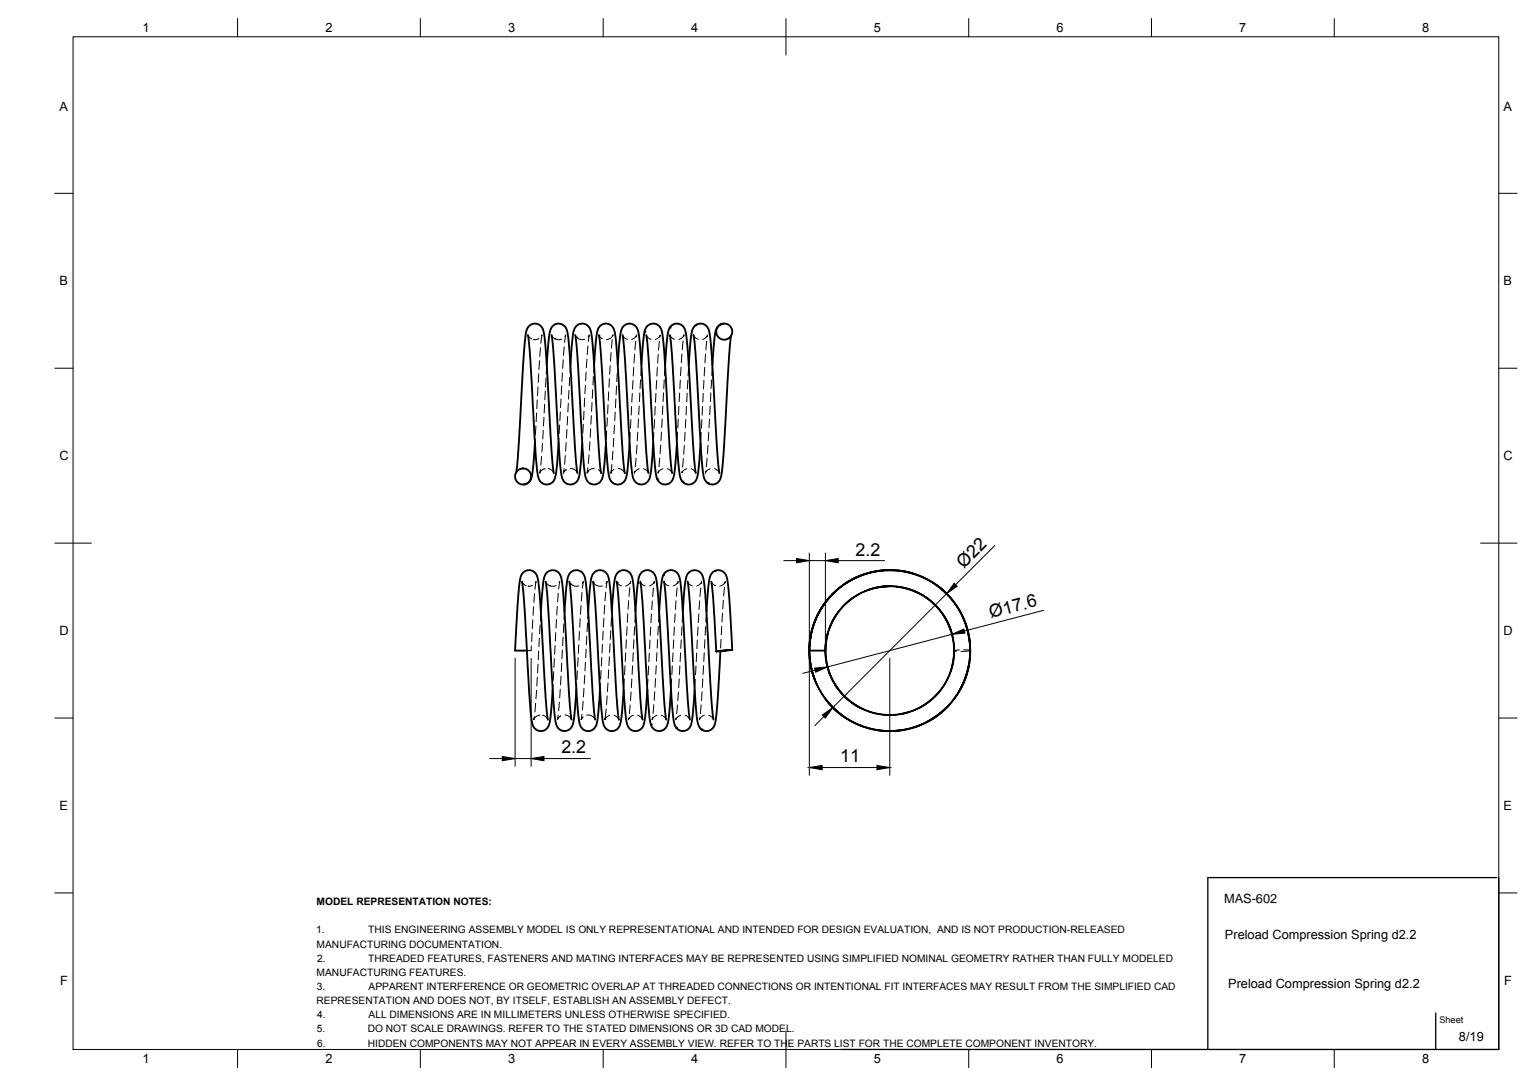
ISO-10303-21;
HEADER;
/* Generated by software containing ST-Developer
 * from STEP Tools, Inc. (www.steptools.com) 
 */

FILE_DESCRIPTION(
/* description */ (''),
/* implementation_level */ '2;1');

FILE_NAME(
/* name */ 'Preload Compression Spring d2.2.step',
/* time_stamp */ '2026-10-15T14:42:47-07:00',
/* author */ (''),
/* organization */ (''),
/* preprocessor_version */ 'ST-DEVELOPER v20.2',
/* originating_system */ 'Autodesk Translation Framework v15.15.0.0',
/* authorisation */ '');

FILE_SCHEMA (('AUTOMOTIVE_DESIGN { 1 0 10303 214 3 1 1 }'));
ENDSEC;

DATA;
#10=MECHANICAL_DESIGN_GEOMETRIC_PRESENTATION_REPRESENTATION('',(#240),#85789);
#204=SHAPE_REPRESENTATION_RELATIONSHIP('SRR','None',#85869,#222);
#222=ADVANCED_BREP_SHAPE_REPRESENTATION('',(#258),#85777);
#240=STYLED_ITEM('',(#85968),#258);
#258=MANIFOLD_SOLID_BREP('Body1',#9887);
#383=B_SPLINE_SURFACE_WITH_KNOTS('',3,3,((#76038,#76039,#76040,#76041,#76042,
#76043,#76044,#76045,#76046,#76047,#76048,#76049,#76050,#76051,#76052,#76053,
#76054,#76055,#76056,#76057,#76058,#76059,#76060,#76061,#76062,#76063,#76064,
#76065,#76066,#76067,#76068,#76069,#76070,#76071,#76072,#76073,#76074,#76075,
#76076,#76077,#76078,#76079,#76080,#76081,#76082,#76083,#76084,#76085,#76086,
#76087,#76088,#76089,#76090,#76091,#76092,#76093,#76094,#76095,#76096,#76097,
#76098,#76099,#76100,#76101,#76102,#76103,#76104,#76105,#76106,#76107,#76108,
#76109,#76110,#76111,#76112,#76113,#76114,#76115,#76116,#76117,#76118,#76119,
#76120,#76121,#76122,#76123,#76124,#76125,#76126,#76127,#76128,#76129,#76130,
#76131,#76132,#76133,#76134,#76135,#76136,#76137,#76138,#76139,#76140,#76141,
#76142,#76143,#76144,#76145,#76146,#76147),(#76148,#76149,#76150,#76151,
#76152,#76153,#76154,#76155,#76156,#76157,#76158,#76159,#76160,#76161,#76162,
#76163,#76164,#76165,#76166,#76167,#76168,#76169,#76170,#76171,#76172,#76173,
#76174,#76175,#76176,#76177,#76178,#76179,#76180,#76181,#76182,#76183,#76184,
#76185,#76186,#76187,#76188,#76189,#76190,#76191,#76192,#76193,#76194,#76195,
#76196,#76197,#76198,#76199,#76200,#76201,#76202,#76203,#76204,#76205,#76206,
#76207,#76208,#76209,#76210,#76211,#76212,#76213,#76214,#76215,#76216,#76217,
#76218,#76219,#76220,#76221,#76222,#76223,#76224,#76225,#76226,#76227,#76228,
#76229,#76230,#76231,#76232,#76233,#76234,#76235,#76236,#76237,#76238,#76239,
#76240,#76241,#76242,#76243,#76244,#76245,#76246,#76247,#76248,#76249,#76250,
#76251,#76252,#76253,#76254,#76255,#76256,#76257),(#76258,#76259,#76260,
#76261,#76262,#76263,#76264,#76265,#76266,#76267,#76268,#76269,#76270,#76271,
#76272,#76273,#76274,#76275,#76276,#76277,#76278,#76279,#76280,#76281,#76282,
#76283,#76284,#76285,#76286,#76287,#76288,#76289,#76290,#76291,#76292,#76293,
#76294,#76295,#76296,#76297,#76298,#76299,#76300,#76301,#76302,#76303,#76304,
#76305,#76306,#76307,#76308,#76309,#76310,#76311,#76312,#76313,#76314,#76315,
#76316,#76317,#76318,#76319,#76320,#76321,#76322,#76323,#76324,#76325,#76326,
#76327,#76328,#76329,#76330,#76331,#76332,#76333,#76334,#76335,#76336,#76337,
#76338,#76339,#76340,#76341,#76342,#76343,#76344,#76345,#76346,#76347,#76348,
#76349,#76350,#76351,#76352,#76353,#76354,#76355,#76356,#76357,#76358,#76359,
#76360,#76361,#76362,#76363,#76364,#76365,#76366,#76367),(#76368,#76369,
#76370,#76371,#76372,#76373,#76374,#76375,#76376,#76377,#76378,#76379,#76380,
#76381,#76382,#76383,#76384,#76385,#76386,#76387,#76388,#76389,#76390,#76391,
#76392,#76393,#76394,#76395,#76396,#76397,#76398,#76399,#76400,#76401,#76402,
#76403,#76404,#76405,#76406,#76407,#76408,#76409,#76410,#76411,#76412,#76413,
#76414,#76415,#76416,#76417,#76418,#76419,#76420,#76421,#76422,#76423,#76424,
#76425,#76426,#76427,#76428,#76429,#76430,#76431,#76432,#76433,#76434,#76435,
#76436,#76437,#76438,#76439,#76440,#76441,#76442,#76443,#76444,#76445,#76446,
#76447,#76448,#76449,#76450,#76451,#76452,#76453,#76454,#76455,#76456,#76457,
#76458,#76459,#76460,#76461,#76462,#76463,#76464,#76465,#76466,#76467,#76468,
#76469,#76470,#76471,#76472,#76473,#76474,#76475,#76476,#76477),(#76478,
#76479,#76480,#76481,#76482,#76483,#76484,#76485,#76486,#76487,#76488,#76489,
#76490,#76491,#76492,#76493,#76494,#76495,#76496,#76497,#76498,#76499,#76500,
#76501,#76502,#76503,#76504,#76505,#76506,#76507,#76508,#76509,#76510,#76511,
#76512,#76513,#76514,#76515,#76516,#76517,#76518,#76519,#76520,#76521,#76522,
#76523,#76524,#76525,#76526,#76527,#76528,#76529,#76530,#76531,#76532,#76533,
#76534,#76535,#76536,#76537,#76538,#76539,#76540,#76541,#76542,#76543,#76544,
#76545,#76546,#76547,#76548,#76549,#76550,#76551,#76552,#76553,#76554,#76555,
#76556,#76557,#76558,#76559,#76560,#76561,#76562,#76563,#76564,#76565,#76566,
#76567,#76568,#76569,#76570,#76571,#76572,#76573,#76574,#76575,#76576,#76577,
#76578,#76579,#76580,#76581,#76582,#76583,#76584,#76585,#76586,#76587),
(#76588,#76589,#76590,#76591,#76592,#76593,#76594,#76595,#76596,#76597,
#76598,#76599,#76600,#76601,#76602,#76603,#76604,#76605,#76606,#76607,#76608,
#76609,#76610,#76611,#76612,#76613,#76614,#76615,#76616,#76617,#76618,#76619,
#76620,#76621,#76622,#76623,#76624,#76625,#76626,#76627,#76628,#76629,#76630,
#76631,#76632,#76633,#76634,#76635,#76636,#76637,#76638,#76639,#76640,#76641,
#76642,#76643,#76644,#76645,#76646,#76647,#76648,#76649,#76650,#76651,#76652,
#76653,#76654,#76655,#76656,#76657,#76658,#76659,#76660,#76661,#76662,#76663,
#76664,#76665,#76666,#76667,#76668,#76669,#76670,#76671,#76672,#76673,#76674,
#76675,#76676,#76677,#76678,#76679,#76680,#76681,#76682,#76683,#76684,#76685,
#76686,#76687,#76688,#76689,#76690,#76691,#76692,#76693,#76694,#76695,#76696,
#76697),(#76698,#76699,#76700,#76701,#76702,#76703,#76704,#76705,#76706,
#76707,#76708,#76709,#76710,#76711,#76712,#76713,#76714,#76715,#76716,#76717,
#76718,#76719,#76720,#76721,#76722,#76723,#76724,#76725,#76726,#76727,#76728,
#76729,#76730,#76731,#76732,#76733,#76734,#76735,#76736,#76737,#76738,#76739,
#76740,#76741,#76742,#76743,#76744,#76745,#76746,#76747,#76748,#76749,#76750,
#76751,#76752,#76753,#76754,#76755,#76756,#76757,#76758,#76759,#76760,#76761,
#76762,#76763,#76764,#76765,#76766,#76767,#76768,#76769,#76770,#76771,#76772,
#76773,#76774,#76775,#76776,#76777,#76778,#76779,#76780,#76781,#76782,#76783,
#76784,#76785,#76786,#76787,#76788,#76789,#76790,#76791,#76792,#76793,#76794,
#76795,#76796,#76797,#76798,#76799,#76800,#76801,#76802,#76803,#76804,#76805,
#76806,#76807),(#76808,#76809,#76810,#76811,#76812,#76813,#76814,#76815,
#76816,#76817,#76818,#76819,#76820,#76821,#76822,#76823,#76824,#76825,#76826,
#76827,#76828,#76829,#76830,#76831,#76832,#76833,#76834,#76835,#76836,#76837,
#76838,#76839,#76840,#76841,#76842,#76843,#76844,#76845,#76846,#76847,#76848,
#76849,#76850,#76851,#76852,#76853,#76854,#76855,#76856,#76857,#76858,#76859,
#76860,#76861,#76862,#76863,#76864,#76865,#76866,#76867,#76868,#76869,#76870,
#76871,#76872,#76873,#76874,#76875,#76876,#76877,#76878,#76879,#76880,#76881,
#76882,#76883,#76884,#76885,#76886,#76887,#76888,#76889,#76890,#76891,#76892,
#76893,#76894,#76895,#76896,#76897,#76898,#76899,#76900,#76901,#76902,#76903,
#76904,#76905,#76906,#76907,#76908,#76909,#76910,#76911,#76912,#76913,#76914,
#76915,#76916,#76917),(#76918,#76919,#76920,#76921,#76922,#76923,#76924,
#76925,#76926,#76927,#76928,#76929,#76930,#76931,#76932,#76933,#76934,#76935,
#76936,#76937,#76938,#76939,#76940,#76941,#76942,#76943,#76944,#76945,#76946,
#76947,#76948,#76949,#76950,#76951,#76952,#76953,#76954,#76955,#76956,#76957,
#76958,#76959,#76960,#76961,#76962,#76963,#76964,#76965,#76966,#76967,#76968,
#76969,#76970,#76971,#76972,#76973,#76974,#76975,#76976,#76977,#76978,#76979,
#76980,#76981,#76982,#76983,#76984,#76985,#76986,#76987,#76988,#76989,#76990,
#76991,#76992,#76993,#76994,#76995,#76996,#76997,#76998,#76999,#77000,#77001,
#77002,#77003,#77004,#77005,#77006,#77007,#77008,#77009,#77010,#77011,#77012,
#77013,#77014,#77015,#77016,#77017,#77018,#77019,#77020,#77021,#77022,#77023,
#77024,#77025,#77026,#77027),(#77028,#77029,#77030,#77031,#77032,#77033,
#77034,#77035,#77036,#77037,#77038,#77039,#77040,#77041,#77042,#77043,#77044,
#77045,#77046,#77047,#77048,#77049,#77050,#77051,#77052,#77053,#77054,#77055,
#77056,#77057,#77058,#77059,#77060,#77061,#77062,#77063,#77064,#77065,#77066,
#77067,#77068,#77069,#77070,#77071,#77072,#77073,#77074,#77075,#77076,#77077,
#77078,#77079,#77080,#77081,#77082,#77083,#77084,#77085,#77086,#77087,#77088,
#77089,#77090,#77091,#77092,#77093,#77094,#77095,#77096,#77097,#77098,#77099,
#77100,#77101,#77102,#77103,#77104,#77105,#77106,#77107,#77108,#77109,#77110,
#77111,#77112,#77113,#77114,#77115,#77116,#77117,#77118,#77119,#77120,#77121,
#77122,#77123,#77124,#77125,#77126,#77127,#77128,#77129,#77130,#77131,#77132,
#77133,#77134,#77135,#77136,#77137)),.UNSPECIFIED.,.T.,.F.,.F.,(4,1,1,1,
1,1,1,4),(4,1,1,1,1,1,1,1,1,1,1,1,1,1,1,1,1,1,1,1,1,1,1,1,1,1,1,1,1,1,1,
1,1,1,1,1,1,1,1,1,1,1,1,1,1,1,1,1,1,1,1,1,1,1,1,1,1,1,1,1,1,1,1,1,1,1,1,
1,1,1,1,1,1,1,1,1,1,1,1,1,1,1,1,1,1,1,1,1,1,1,1,1,1,1,1,1,1,1,1,1,1,1,1,
1,1,1,1,4),(-3.14159265358979,-2.24399475256414,-1.34639685153848,-0.448798950512828,
0.448798950512828,1.34639685153848,2.24399475256414,3.14159265358979),(0.,
0.00446428571428571,0.00892857142857143,0.0178571428571429,0.0267857142857143,
0.0357142857142857,0.0446428571428571,0.0535714285714286,0.0625,0.0714285714285714,
0.0803571428571428,0.0892857142857143,0.0982142857142857,0.107142857142857,
0.116071428571429,0.125,0.133928571428571,0.142857142857143,0.154761904761905,
0.166666666666667,0.178571428571429,0.18452380952381,0.19047619047619,0.196428571428571,
0.202380952380952,0.214285714285714,0.222222222222222,0.23015873015873,
0.238095238095238,0.244047619047619,0.25,0.261904761904762,0.273809523809524,
0.285714285714286,0.297619047619048,0.30952380952381,0.321428571428571,
0.333333333333333,0.341269841269841,0.349206349206349,0.357142857142857,
0.365079365079365,0.373015873015873,0.380952380952381,0.392857142857143,
0.404761904761905,0.416666666666667,0.428571428571429,0.44047619047619,
0.452380952380952,0.46031746031746,0.468253968253968,0.472222222222222,
0.476190476190476,0.486772486772487,0.492063492063492,0.5,0.507936507936508,
0.515873015873016,0.523809523809524,0.535714285714286,0.547619047619048,
0.55952380952381,0.571428571428571,0.583333333333333,0.595238095238095,
0.607142857142857,0.619047619047619,0.626984126984127,0.634920634920635,
0.642857142857143,0.650793650793651,0.658730158730159,0.666666666666667,
0.674603174603175,0.682539682539683,0.69047619047619,0.702380952380952,
0.714285714285714,0.726190476190476,0.738095238095238,0.75,0.761904761904762,
0.773809523809524,0.785714285714286,0.797619047619047,0.809523809523809,
0.821428571428571,0.833333333333333,0.845238095238095,0.857142857142857,
0.866071428571429,0.875,0.883928571428571,0.892857142857143,0.901785714285714,
0.910714285714286,0.919642857142857,0.928571428571429,0.9375,0.946428571428571,
0.955357142857143,0.964285714285714,0.973214285714286,0.982142857142857,
0.991071428571429,0.995535714285714,1.),.UNSPECIFIED.);
#905=B_SPLINE_CURVE_WITH_KNOTS('',3,(#77139,#77140,#77141,#77142,#77143,
#77144,#77145,#77146,#77147,#77148,#77149,#77150,#77151,#77152,#77153,#77154,
#77155,#77156,#77157,#77158,#77159,#77160,#77161,#77162,#77163,#77164,#77165,
#77166,#77167,#77168,#77169,#77170,#77171,#77172,#77173,#77174,#77175,#77176),
 .UNSPECIFIED.,.T.,.F.,(4,2,2,2,2,2,2,2,2,2,2,2,2,2,2,2,2,2,4),(-0.605125399548974,
-0.601986519691417,-0.572296417272211,-0.544506901286991,-0.51205526449825,
-0.473980307125887,-0.436263250016685,-0.397515325089208,-0.367226247639718,
-0.338720455098409,-0.30995049023698,-0.27886558943038,-0.238746391927005,
-0.193651773165657,-0.137323097666455,-0.0888290194031273,-0.0473891574083154,
-0.00368586125467713,0.),.UNSPECIFIED.);
#906=B_SPLINE_CURVE_WITH_KNOTS('',3,(#77178,#77179,#77180,#77181,#77182,
#77183,#77184,#77185,#77186,#77187,#77188,#77189,#77190,#77191,#77192,#77193,
#77194,#77195,#77196,#77197,#77198,#77199,#77200,#77201,#77202,#77203,#77204,
#77205,#77206,#77207,#77208,#77209,#77210,#77211,#77212,#77213,#77214,#77215,
#77216,#77217,#77218,#77219,#77220,#77221,#77222,#77223,#77224,#77225,#77226,
#77227,#77228,#77229,#77230,#77231,#77232,#77233,#77234,#77235,#77236,#77237,
#77238,#77239,#77240,#77241,#77242,#77243,#77244,#77245,#77246,#77247,#77248,
#77249,#77250,#77251,#77252,#77253,#77254,#77255,#77256,#77257,#77258,#77259,
#77260,#77261,#77262,#77263,#77264,#77265,#77266,#77267,#77268,#77269,#77270,
#77271,#77272,#77273,#77274,#77275,#77276,#77277,#77278,#77279,#77280,#77281,
#77282,#77283,#77284,#77285,#77286,#77287),.UNSPECIFIED.,.F.,.F.,(4,1,1,
1,1,1,1,1,1,1,1,1,1,1,1,1,1,1,1,1,1,1,1,1,1,1,1,1,1,1,1,1,1,1,1,1,1,1,1,
1,1,1,1,1,1,1,1,1,1,1,1,1,1,1,1,1,1,1,1,1,1,1,1,1,1,1,1,1,1,1,1,1,1,1,1,
1,1,1,1,1,1,1,1,1,1,1,1,1,1,1,1,1,1,1,1,1,1,1,1,1,1,1,1,1,1,1,1,4),(0.,
0.00446428571428571,0.00892857142857143,0.0178571428571429,0.0267857142857143,
0.0357142857142857,0.0446428571428571,0.0535714285714286,0.0625,0.0714285714285714,
0.0803571428571428,0.0892857142857143,0.0982142857142857,0.107142857142857,
0.116071428571429,0.125,0.133928571428571,0.142857142857143,0.154761904761905,
0.166666666666667,0.178571428571429,0.18452380952381,0.19047619047619,0.196428571428571,
0.202380952380952,0.214285714285714,0.222222222222222,0.23015873015873,
0.238095238095238,0.244047619047619,0.25,0.261904761904762,0.273809523809524,
0.285714285714286,0.297619047619048,0.30952380952381,0.321428571428571,
0.333333333333333,0.341269841269841,0.349206349206349,0.357142857142857,
0.365079365079365,0.373015873015873,0.380952380952381,0.392857142857143,
0.404761904761905,0.416666666666667,0.428571428571429,0.44047619047619,
0.452380952380952,0.46031746031746,0.468253968253968,0.472222222222222,
0.476190476190476,0.486772486772487,0.492063492063492,0.5,0.507936507936508,
0.515873015873016,0.523809523809524,0.535714285714286,0.547619047619048,
0.55952380952381,0.571428571428571,0.583333333333333,0.595238095238095,
0.607142857142857,0.619047619047619,0.626984126984127,0.634920634920635,
0.642857142857143,0.650793650793651,0.658730158730159,0.666666666666667,
0.674603174603175,0.682539682539683,0.69047619047619,0.702380952380952,
0.714285714285714,0.726190476190476,0.738095238095238,0.75,0.761904761904762,
0.773809523809524,0.785714285714286,0.797619047619047,0.809523809523809,
0.821428571428571,0.833333333333333,0.845238095238095,0.857142857142857,
0.866071428571429,0.875,0.883928571428571,0.892857142857143,0.901785714285714,
0.910714285714286,0.919642857142857,0.928571428571429,0.9375,0.946428571428571,
0.955357142857143,0.964285714285714,0.973214285714286,0.982142857142857,
0.991071428571429,0.995535714285714,1.),.UNSPECIFIED.);
#907=B_SPLINE_CURVE_WITH_KNOTS('',3,(#77288,#77289,#77290,#77291,#77292,
#77293,#77294,#77295,#77296,#77297,#77298,#77299,#77300,#77301,#77302,#77303,
#77304,#77305,#77306,#77307,#77308,#77309,#77310,#77311,#77312,#77313,#77314,
#77315,#77316,#77317,#77318,#77319,#77320,#77321,#77322,#77323,#77324,#77325),
 .UNSPECIFIED.,.T.,.F.,(4,2,2,2,2,2,2,2,2,2,2,2,2,2,2,2,2,2,4),(-0.605125399680566,
-0.601986519826148,-0.572296417399655,-0.544506901407513,-0.512055264610774,
-0.473980307229046,-0.436263250110675,-0.397515325173783,-0.367226247717055,
-0.338720455168909,-0.309950490300473,-0.278865589486237,-0.238746391973086,
-0.1936517732017,-0.137323097692225,-0.0888290194200642,-0.0473891574177423,
-0.00368586125594956,0.),.UNSPECIFIED.);
#1110=PLANE('',#10563);
#1111=PLANE('',#10564);
#2712=FACE_OUTER_BOUND('',#3276,.T.);
#2713=FACE_OUTER_BOUND('',#3277,.T.);
#2714=FACE_OUTER_BOUND('',#3278,.T.);
#3276=EDGE_LOOP('',(#8405,#8406,#8407,#8408));
#3277=EDGE_LOOP('',(#8409));
#3278=EDGE_LOOP('',(#8410));
#4601=VERTEX_POINT('',#77138);
#4602=VERTEX_POINT('',#77177);
#5930=EDGE_CURVE('',#4601,#4601,#905,.T.);
#5931=EDGE_CURVE('',#4601,#4602,#906,.T.);
#5932=EDGE_CURVE('',#4602,#4602,#907,.T.);
#8405=ORIENTED_EDGE('',*,*,#5930,.T.);
#8406=ORIENTED_EDGE('',*,*,#5931,.T.);
#8407=ORIENTED_EDGE('',*,*,#5932,.F.);
#8408=ORIENTED_EDGE('',*,*,#5931,.F.);
#8409=ORIENTED_EDGE('',*,*,#5932,.T.);
#8410=ORIENTED_EDGE('',*,*,#5930,.F.);
#9690=ADVANCED_FACE('',(#2712),#383,.T.);
#9691=ADVANCED_FACE('',(#2713),#1110,.T.);
#9692=ADVANCED_FACE('',(#2714),#1111,.F.);
#9887=CLOSED_SHELL('',(#9690,#9691,#9692));
#10562=AXIS2_PLACEMENT_3D('',#76037,#12217,#12218);
#10563=AXIS2_PLACEMENT_3D('',#77326,#12219,#12220);
#10564=AXIS2_PLACEMENT_3D('',#77327,#12221,#12222);
#12217=DIRECTION('axis',(0.,0.,1.));
#12218=DIRECTION('refdir',(1.,0.,0.));
#12219=DIRECTION('center_axis',(-0.0185160100832464,-0.994867197984037,
0.0994807305260099));
#12220=DIRECTION('ref_axis',(0.933205561217733,0.0185160101174801,0.358865626497753));
#12221=DIRECTION('center_axis',(0.,1.,0.));
#12222=DIRECTION('ref_axis',(1.,0.,0.));
#76037=CARTESIAN_POINT('',(0.,0.,0.));
#76038=CARTESIAN_POINT('Ctrl Pts',(0.88,2.1,9.525));
#76039=CARTESIAN_POINT('Ctrl Pts',(0.879914606625585,2.17110785049955,9.52865476385635));
#76040=CARTESIAN_POINT('Ctrl Pts',(0.863232117186907,2.3095104036224,9.53591397312323));
#76041=CARTESIAN_POINT('Ctrl Pts',(0.7646146646842,2.57432753790838,9.55048599717583));
#76042=CARTESIAN_POINT('Ctrl Pts',(0.52875066403414,2.8457083400553,9.56867094599734));
#76043=CARTESIAN_POINT('Ctrl Pts',(0.127238756664634,3.00552936974926,9.59051359518968));
#76044=CARTESIAN_POINT('Ctrl Pts',(-0.302716205619033,2.96306288294985,
9.61235380295566));
#76045=CARTESIAN_POINT('Ctrl Pts',(-0.665427657999688,2.72799341501097,
9.63420407641812));
#76046=CARTESIAN_POINT('Ctrl Pts',(-0.879826065415376,2.3524940033895,9.65606121698024));
#76047=CARTESIAN_POINT('Ctrl Pts',(-0.89799221853441,1.92029343459682,9.67792905414005));
#76048=CARTESIAN_POINT('Ctrl Pts',(-0.715657796510551,1.52775201761214,
9.69980826165769));
#76049=CARTESIAN_POINT('Ctrl Pts',(-0.37329244035757,1.26252484692041,9.72170089413125));
#76050=CARTESIAN_POINT('Ctrl Pts',(0.0529042162174613,1.18397194405211,
9.7436083723133));
#76051=CARTESIAN_POINT('Ctrl Pts',(0.467926525737336,1.30987826775351,9.76553239226868));
#76052=CARTESIAN_POINT('Ctrl Pts',(0.77911594458734,1.61250328722602,9.78747453406851));
#76053=CARTESIAN_POINT('Ctrl Pts',(0.916833254715888,2.02450810034898,9.8094364412056));
#76054=CARTESIAN_POINT('Ctrl Pts',(0.84999015619955,2.45432327019144,9.83141968646686));
#76055=CARTESIAN_POINT('Ctrl Pts',(0.593134887517594,2.80556810401153,9.85342584950507));
#76056=CARTESIAN_POINT('Ctrl Pts',(0.159785468035136,3.02235194398505,9.87790429996245));
#76057=CARTESIAN_POINT('Ctrl Pts',(-0.382738476891779,2.97204316801605,
9.90486768286448));
#76058=CARTESIAN_POINT('Ctrl Pts',(-0.827943575417754,2.57464859578558,
9.93433214776037));
#76059=CARTESIAN_POINT('Ctrl Pts',(-0.928540642244484,2.0879125901631,9.95893043030863));
#76060=CARTESIAN_POINT('Ctrl Pts',(-0.82506221727755,1.71823863855703,9.97863755083128));
#76061=CARTESIAN_POINT('Ctrl Pts',(-0.665238898770628,1.47861418311032,
9.99343255715118));
#76062=CARTESIAN_POINT('Ctrl Pts',(-0.438025190317537,1.3012081221325,10.0082426633322));
#76063=CARTESIAN_POINT('Ctrl Pts',(-0.0759140953759721,1.16989403941721,
10.0280101634631));
#76064=CARTESIAN_POINT('Ctrl Pts',(0.353590617267489,1.22647296601624,10.0494595111079));
#76065=CARTESIAN_POINT('Ctrl Pts',(0.71282299611785,1.50640456177768,10.0726022736917));
#76066=CARTESIAN_POINT('Ctrl Pts',(0.895311256816217,1.85157831854142,10.0924697020734));
#76067=CARTESIAN_POINT('Ctrl Pts',(0.917661293713379,2.20976194577009,10.1107106042816));
#76068=CARTESIAN_POINT('Ctrl Pts',(0.819212469046223,2.51761130734418,10.127317066638));
#76069=CARTESIAN_POINT('Ctrl Pts',(0.591924394917487,2.83289082559773,10.1472698428113));
#76070=CARTESIAN_POINT('Ctrl Pts',(0.141288805504938,3.06103897732418,10.172258699084));
#76071=CARTESIAN_POINT('Ctrl Pts',(-0.458527011040082,2.95925151709148,
10.2023249565719));
#76072=CARTESIAN_POINT('Ctrl Pts',(-0.88162766536303,2.52027411449529,10.2324736532743));
#76073=CARTESIAN_POINT('Ctrl Pts',(-0.961653185964405,1.91393657438503,
10.2627077273853));
#76074=CARTESIAN_POINT('Ctrl Pts',(-0.665231767857691,1.37715957803001,
10.2930297792945));
#76075=CARTESIAN_POINT('Ctrl Pts',(-0.105988685338195,1.12026073865136,
10.3234425669733));
#76076=CARTESIAN_POINT('Ctrl Pts',(0.430538820721984,1.23255710504194,10.3505590141325));
#76077=CARTESIAN_POINT('Ctrl Pts',(0.777157271318668,1.54704609431923,10.3743479205533));
#76078=CARTESIAN_POINT('Ctrl Pts',(0.937973646848606,1.91510656924282,10.3947816504623));
#76079=CARTESIAN_POINT('Ctrl Pts',(0.932931736507626,2.31778957988939,10.4152592321293));
#76080=CARTESIAN_POINT('Ctrl Pts',(0.762578582228501,2.68366310973811,10.4357813746755));
#76081=CARTESIAN_POINT('Ctrl Pts',(0.455963235969408,2.94715653506223,10.4563486739678));
#76082=CARTESIAN_POINT('Ctrl Pts',(0.00240142086611935,3.08166579400621,
10.480397254692));
#76083=CARTESIAN_POINT('Ctrl Pts',(-0.538455390507358,2.94820992747045,
10.5079586157699));
#76084=CARTESIAN_POINT('Ctrl Pts',(-0.940666416691817,2.46401744657124,
10.5390713811047));
#76085=CARTESIAN_POINT('Ctrl Pts',(-0.976029443563649,1.83335883304997,
10.5702921359498));
#76086=CARTESIAN_POINT('Ctrl Pts',(-0.629306856593687,1.30317046301086,
10.6016225477596));
#76087=CARTESIAN_POINT('Ctrl Pts',(-0.0328763589810331,1.08144514613719,
10.6330641573791));
#76088=CARTESIAN_POINT('Ctrl Pts',(0.511901871764286,1.23876013099839,10.6611123163153));
#76089=CARTESIAN_POINT('Ctrl Pts',(0.845208777494887,1.59002857501027,10.6857282761483));
#76090=CARTESIAN_POINT('Ctrl Pts',(0.959937391714928,1.91692164410815,10.7033535735637));
#76091=CARTESIAN_POINT('Ctrl Pts',(0.964709509971458,2.19002072343591,10.7174794574177));
#76092=CARTESIAN_POINT('Ctrl Pts',(0.903969607200192,2.50338072207659,10.7339796596208));
#76093=CARTESIAN_POINT('Ctrl Pts',(0.708976511873778,2.79903473649909,10.7516978643424));
#76094=CARTESIAN_POINT('Ctrl Pts',(0.359111666410103,3.02058677865832,10.7730116718645));
#76095=CARTESIAN_POINT('Ctrl Pts',(-0.0055195068732309,3.09939687665217,
10.7919958841582));
#76096=CARTESIAN_POINT('Ctrl Pts',(-0.417331250225881,3.01093271757532,
10.8134054790171));
#76097=CARTESIAN_POINT('Ctrl Pts',(-0.756608961158023,2.76032613000462,
10.8348676292604));
#76098=CARTESIAN_POINT('Ctrl Pts',(-0.998865593098056,2.33000290793379,
10.8599683150449));
#76099=CARTESIAN_POINT('Ctrl Pts',(-0.988791187924089,1.74845036869023,
10.8887429491342));
#76100=CARTESIAN_POINT('Ctrl Pts',(-0.588714669350558,1.22669384301482,
10.9212338011637));
#76101=CARTESIAN_POINT('Ctrl Pts',(0.044909234496707,1.04388405761621,10.9538443040117));
#76102=CARTESIAN_POINT('Ctrl Pts',(0.665762350574508,1.27382859359802,10.9865746011287));
#76103=CARTESIAN_POINT('Ctrl Pts',(1.02994927065475,1.82963242200099,11.0194247010519));
#76104=CARTESIAN_POINT('Ctrl Pts',(0.99292771913683,2.49532007970257,11.0523944801788));
#76105=CARTESIAN_POINT('Ctrl Pts',(0.566047404042377,3.01118540039736,11.0854836852924));
#76106=CARTESIAN_POINT('Ctrl Pts',(-0.0131656805453273,3.1545072720966,
11.1150021335127));
#76107=CARTESIAN_POINT('Ctrl Pts',(-0.501834747536299,3.00971245930524,
11.1409075995603));
#76108=CARTESIAN_POINT('Ctrl Pts',(-0.833654637909307,2.72466132918788,
11.1631647757637));
#76109=CARTESIAN_POINT('Ctrl Pts',(-1.01904932840502,2.32688792491809,11.1854742337572));
#76110=CARTESIAN_POINT('Ctrl Pts',(-1.0247320303861,1.8873087550975,11.2078357472338));
#76111=CARTESIAN_POINT('Ctrl Pts',(-0.848433071641297,1.48323440703255,
11.2302490424206));
#76112=CARTESIAN_POINT('Ctrl Pts',(-0.5209916303453,1.18686010809674,11.2527138516101));
#76113=CARTESIAN_POINT('Ctrl Pts',(-0.0994474829318688,1.05086828612434,
11.2752298585268));
#76114=CARTESIAN_POINT('Ctrl Pts',(0.341286571712092,1.10081439784123,11.297796723956));
#76115=CARTESIAN_POINT('Ctrl Pts',(0.787934060544661,1.36522529701193,11.3241836591263));
#76116=CARTESIAN_POINT('Ctrl Pts',(1.08440822726537,1.89981767692546,11.3544236935599));
#76117=CARTESIAN_POINT('Ctrl Pts',(0.99437189083192,2.58466520846377,11.3885550724356));
#76118=CARTESIAN_POINT('Ctrl Pts',(0.51422832678732,3.08343949927552,11.4227963300144));
#76119=CARTESIAN_POINT('Ctrl Pts',(-0.170956362315584,3.20042729316684,
11.4571457685877));
#76120=CARTESIAN_POINT('Ctrl Pts',(-0.792809143568463,2.88603885152724,
11.49160167588));
#76121=CARTESIAN_POINT('Ctrl Pts',(-1.10815562220614,2.26212033857722,11.5261621918766));
#76122=CARTESIAN_POINT('Ctrl Pts',(-0.990980784814367,1.57098681332194,
11.5608252913622));
#76123=CARTESIAN_POINT('Ctrl Pts',(-0.484736723033935,1.08260154598769,
11.5955889188738));
#76124=CARTESIAN_POINT('Ctrl Pts',(0.214307763377102,0.991032096532327,
11.6304507824074));
#76125=CARTESIAN_POINT('Ctrl Pts',(0.833298379906107,1.33271197734595,11.6654086518246));
#76126=CARTESIAN_POINT('Ctrl Pts',(1.12908711130714,1.97705558535849,11.7004600148669));
#76127=CARTESIAN_POINT('Ctrl Pts',(0.984170425255086,2.67277304384029,11.7356024461146));
#76128=CARTESIAN_POINT('Ctrl Pts',(0.452808643636702,3.14802102155422,11.7708333087139));
#76129=CARTESIAN_POINT('Ctrl Pts',(-0.198836507924274,3.20872213800758,
11.8032068201948));
#76130=CARTESIAN_POINT('Ctrl Pts',(-0.720833985617695,2.9475724124579,11.8326976979388));
#76131=CARTESIAN_POINT('Ctrl Pts',(-1.03122512713103,2.52323917223077,11.8592848682016));
#76132=CARTESIAN_POINT('Ctrl Pts',(-1.11221371795246,2.00254397936835,11.8859162010712));
#76133=CARTESIAN_POINT('Ctrl Pts',(-0.944978677865563,1.50212478400673,
11.9125904181942));
#76134=CARTESIAN_POINT('Ctrl Pts',(-0.566096651435205,1.13364169683645,
11.9393062323883));
#76135=CARTESIAN_POINT('Ctrl Pts',(-0.0596069971212731,0.97996909355213,
11.966062281935));
#76136=CARTESIAN_POINT('Ctrl Pts',(0.461675051948685,1.07603593590851,11.9928572469173));
#76137=CARTESIAN_POINT('Ctrl Pts',(0.88129231323125,1.40110770643291,12.0196896905075));
#76138=CARTESIAN_POINT('Ctrl Pts',(1.10519737818586,1.88315811002375,12.0465583931276));
#76139=CARTESIAN_POINT('Ctrl Pts',(1.08283365883886,2.41488670097258,12.0734615789711));
#76140=CARTESIAN_POINT('Ctrl Pts',(0.818591168747924,2.87760074176854,12.100398642491));
#76141=CARTESIAN_POINT('Ctrl Pts',(0.370893737846914,3.16774776724325,12.1273662612715));
#76142=CARTESIAN_POINT('Ctrl Pts',(-0.160578831483255,3.22009488317826,
12.154367120808));
#76143=CARTESIAN_POINT('Ctrl Pts',(-0.657438304412148,3.02243699025829,
12.181390412703));
#76144=CARTESIAN_POINT('Ctrl Pts',(-0.949764066307816,2.68573447988004,
12.2039450357004));
#76145=CARTESIAN_POINT('Ctrl Pts',(-1.07182425162092,2.35796849387404,12.2219800536891));
#76146=CARTESIAN_POINT('Ctrl Pts',(-1.09256785760649,2.18550272007321,12.2310256553714));
#76147=CARTESIAN_POINT('Ctrl Pts',(-1.09265261173395,2.09796323888708,12.2355247810852));
#76148=CARTESIAN_POINT('Ctrl Pts',(0.88,2.1,9.55791192303761));
#76149=CARTESIAN_POINT('Ctrl Pts',(0.879783916285541,2.17106190544998,9.56156549634868));
#76150=CARTESIAN_POINT('Ctrl Pts',(0.862819487639945,2.30936028696044,9.56882270408062));
#76151=CARTESIAN_POINT('Ctrl Pts',(0.763769645522231,2.57374536624056,9.58338184659129));
#76152=CARTESIAN_POINT('Ctrl Pts',(0.527681439909107,2.84421258618503,9.60154403506069));
#76153=CARTESIAN_POINT('Ctrl Pts',(0.126836189332554,3.00282054305338,9.6233360843192));
#76154=CARTESIAN_POINT('Ctrl Pts',(-0.301578089003487,2.9596327314869,9.64510671305593));
#76155=CARTESIAN_POINT('Ctrl Pts',(-0.662248104445556,2.72485823025643,
9.66686668449843));
#76156=CARTESIAN_POINT('Ctrl Pts',(-0.87477101414986,2.35090800902427,9.68861370251383));
#76157=CARTESIAN_POINT('Ctrl Pts',(-0.891962086690084,1.92134378925048,
9.71035132236448));
#76158=CARTESIAN_POINT('Ctrl Pts',(-0.71013501547485,1.53195117584763,9.73208047576603));
#76159=CARTESIAN_POINT('Ctrl Pts',(-0.369972269812193,1.2695301574022,9.75380324748816));
#76160=CARTESIAN_POINT('Ctrl Pts',(0.0525992830413849,1.19253118829567,
9.77552119527361));
#76161=CARTESIAN_POINT('Ctrl Pts',(0.463319878103491,1.31804354326137,9.79723612745198));
#76162=CARTESIAN_POINT('Ctrl Pts',(0.770594784068131,1.61807714145974,9.81894973497212));
#76163=CARTESIAN_POINT('Ctrl Pts',(0.90590391628519,2.02562383372829,9.84066384510364));
#76164=CARTESIAN_POINT('Ctrl Pts',(0.839026217634196,2.44999742219886,9.86238006152402));
#76165=CARTESIAN_POINT('Ctrl Pts',(0.584857943541199,2.79609540610752,9.88410036302005));
#76166=CARTESIAN_POINT('Ctrl Pts',(0.15715540696274,3.00896823215133,9.90823975031835));
#76167=CARTESIAN_POINT('Ctrl Pts',(-0.377152993385563,2.95829410746318,
9.93480658955309));
#76168=CARTESIAN_POINT('Ctrl Pts',(-0.814397042063615,2.56634291336892,
9.96380668194593));
#76169=CARTESIAN_POINT('Ctrl Pts',(-0.912281798203633,2.08773618372905,
9.9879885560003));
#76170=CARTESIAN_POINT('Ctrl Pts',(-0.80994027967792,1.72488593264374,10.007344749781));
#76171=CARTESIAN_POINT('Ctrl Pts',(-0.652597501593231,1.48997710639104,
10.0218694825692));
#76172=CARTESIAN_POINT('Ctrl Pts',(-0.429334265664847,1.31636286686092,
10.036401726932));
#76173=CARTESIAN_POINT('Ctrl Pts',(-0.0739971908554309,1.18829325899891,
10.0557871102574));
#76174=CARTESIAN_POINT('Ctrl Pts',(0.346806406792938,1.24460770613069,10.0768146985648));
#76175=CARTESIAN_POINT('Ctrl Pts',(0.697974642411667,1.51937892964619,10.0994750183564));
#76176=CARTESIAN_POINT('Ctrl Pts',(0.87586983164938,1.85746669220029,10.1189161511382));
#76177=CARTESIAN_POINT('Ctrl Pts',(0.897034042189538,2.20777551093713,10.1367564439922));
#76178=CARTESIAN_POINT('Ctrl Pts',(0.800234096584245,2.5084630157536,10.152988370211));
#76179=CARTESIAN_POINT('Ctrl Pts',(0.577596139139017,2.81603174879275,10.1724819296167));
#76180=CARTESIAN_POINT('Ctrl Pts',(0.137179583427464,3.03788753933788,10.1968844302235));
#76181=CARTESIAN_POINT('Ctrl Pts',(-0.447719726782846,2.93741039885078,
10.2262174469579));
#76182=CARTESIAN_POINT('Ctrl Pts',(-0.8592452583341,2.50872159304617,10.2556077729931));
#76183=CARTESIAN_POINT('Ctrl Pts',(-0.935997001543472,1.91804036079765,
10.2850576889373));
#76184=CARTESIAN_POINT('Ctrl Pts',(-0.646471737706749,1.3962267816677,10.3145716941238));
#76185=CARTESIAN_POINT('Ctrl Pts',(-0.102097088466362,1.14747264463815,
10.3441525825305));
#76186=CARTESIAN_POINT('Ctrl Pts',(0.419131076191686,1.25764685588435,10.3705107921544));
#76187=CARTESIAN_POINT('Ctrl Pts',(0.755233370608568,1.56377441619041,10.3936200727939));
#76188=CARTESIAN_POINT('Ctrl Pts',(0.910698712173214,1.92145284521483,10.4134626290806));
#76189=CARTESIAN_POINT('Ctrl Pts',(0.905060795811563,2.3122898350333,10.433339759045));
#76190=CARTESIAN_POINT('Ctrl Pts',(0.739099621706325,2.66695860331452,10.453252117855));
#76191=CARTESIAN_POINT('Ctrl Pts',(0.441230372512847,2.92195825542685,10.4732014482075));
#76192=CARTESIAN_POINT('Ctrl Pts',(0.00121674788033055,3.05154102121814,
10.4965196435521));
#76193=CARTESIAN_POINT('Ctrl Pts',(-0.522748489859997,2.92119140764988,
10.5232357617401));
#76194=CARTESIAN_POINT('Ctrl Pts',(-0.911497386825926,2.45137002542038,
10.5533776932785));
#76195=CARTESIAN_POINT('Ctrl Pts',(-0.944589337394057,1.84057261493696,
10.5836150456035));
#76196=CARTESIAN_POINT('Ctrl Pts',(-0.607970601887274,1.32795366098775,
10.6139463426483));
#76197=CARTESIAN_POINT('Ctrl Pts',(-0.0303722616549957,1.11446027835103,
10.6443758271437));
#76198=CARTESIAN_POINT('Ctrl Pts',(0.496414421501777,1.26764280902697,10.6715139458982));
#76199=CARTESIAN_POINT('Ctrl Pts',(0.818195108939898,1.60801290269984,10.6953251867043));
#76200=CARTESIAN_POINT('Ctrl Pts',(0.928577482097722,1.92437513921087,10.7123719721017));
#76201=CARTESIAN_POINT('Ctrl Pts',(0.932712814366555,2.18849028957719,10.7260329283826));
#76202=CARTESIAN_POINT('Ctrl Pts',(0.873425627776733,2.49140923636693,10.7419890654634));
#76203=CARTESIAN_POINT('Ctrl Pts',(0.684360362767623,2.77694456454821,10.7591217708996));
#76204=CARTESIAN_POINT('Ctrl Pts',(0.345706151983871,2.99053966910833,10.779728973541));
#76205=CARTESIAN_POINT('Ctrl Pts',(-0.00695621592430146,3.06609903601776,
10.7980830429247));
#76206=CARTESIAN_POINT('Ctrl Pts',(-0.404919858613662,2.97985927827303,
10.8187806195429));
#76207=CARTESIAN_POINT('Ctrl Pts',(-0.732470914203224,2.73700800230651,
10.8395282778942));
#76208=CARTESIAN_POINT('Ctrl Pts',(-0.965916457583696,2.32059708248666,
10.8637928468312));
#76209=CARTESIAN_POINT('Ctrl Pts',(-0.955180521436829,1.75843199962428,
10.8916085044493));
#76210=CARTESIAN_POINT('Ctrl Pts',(-0.567524852982291,1.25471553979666,
10.9230176634458));
#76211=CARTESIAN_POINT('Ctrl Pts',(0.0453742137555828,1.07904710642372,
10.9545445596419));
#76212=CARTESIAN_POINT('Ctrl Pts',(0.645298788561736,1.30242661576631,10.9861905897209));
#76213=CARTESIAN_POINT('Ctrl Pts',(0.996561212876046,1.84052731934913,11.0179569335076));
#76214=CARTESIAN_POINT('Ctrl Pts',(0.95965217440279,2.48434133424897,11.0498444512395));
#76215=CARTESIAN_POINT('Ctrl Pts',(0.545822723695986,2.98271084435086,11.081854458347));
#76216=CARTESIAN_POINT('Ctrl Pts',(-0.014904284913205,3.12045730942825,
11.1104164211207));
#76217=CARTESIAN_POINT('Ctrl Pts',(-0.487661806414971,2.97950014590718,
11.1354897161336));
#76218=CARTESIAN_POINT('Ctrl Pts',(-0.808440019610243,2.70298642271134,
11.157036944517));
#76219=CARTESIAN_POINT('Ctrl Pts',(-0.987310850925297,2.31750955387077,
11.1786378910855));
#76220=CARTESIAN_POINT('Ctrl Pts',(-0.992098225376437,1.89173243381715,
11.2002962144121));
#76221=CARTESIAN_POINT('Ctrl Pts',(-0.82064376921839,1.5005573687953,11.2220077836223));
#76222=CARTESIAN_POINT('Ctrl Pts',(-0.502851712636325,1.21388588160114,
11.2437762289073));
#76223=CARTESIAN_POINT('Ctrl Pts',(-0.0940215246938652,1.08275155627072,
11.2655990874032));
#76224=CARTESIAN_POINT('Ctrl Pts',(0.333245621813066,1.13189689359355,11.2874794932251));
#76225=CARTESIAN_POINT('Ctrl Pts',(0.766035799756981,1.38907373699405,11.3130716739573));
#76226=CARTESIAN_POINT('Ctrl Pts',(1.05285688105598,1.90823270195865,11.3424078568475));
#76227=CARTESIAN_POINT('Ctrl Pts',(0.964393978317041,2.57292853569788,11.375537780296));
#76228=CARTESIAN_POINT('Ctrl Pts',(0.497259385622897,3.05663886627931,11.408792079458));
#76229=CARTESIAN_POINT('Ctrl Pts',(-0.168799592857434,3.16928654041918,
11.4421680598492));
#76230=CARTESIAN_POINT('Ctrl Pts',(-0.773028708878503,2.86260976094568,
11.4756720319812));
#76231=CARTESIAN_POINT('Ctrl Pts',(-1.07892178246083,2.25506720291879,11.5092937866771));
#76232=CARTESIAN_POINT('Ctrl Pts',(-0.963794044402426,1.58234479055142,
11.5430382284851));
#76233=CARTESIAN_POINT('Ctrl Pts',(-0.469862016813641,1.10729279591243,
11.5768999608508));
#76234=CARTESIAN_POINT('Ctrl Pts',(0.211814495863296,1.019066613562,11.610886222149));
#76235=CARTESIAN_POINT('Ctrl Pts',(0.815201055217733,1.35332341694216,11.6449854463145));
#76236=CARTESIAN_POINT('Ctrl Pts',(1.10303660712102,1.98284539338398,11.6792011961435));
#76237=CARTESIAN_POINT('Ctrl Pts',(0.960427736142072,2.66238095948827,11.7135308697322));
#76238=CARTESIAN_POINT('Ctrl Pts',(0.440172394309644,3.12630195146006,11.7479736075752));
#76239=CARTESIAN_POINT('Ctrl Pts',(-0.197583641464606,3.18475546487694,
11.7796461293911));
#76240=CARTESIAN_POINT('Ctrl Pts',(-0.708367033845548,2.92823812698208,
11.8085215502503));
#76241=CARTESIAN_POINT('Ctrl Pts',(-1.01186730074176,2.51199019692748,11.8345688321747));
#76242=CARTESIAN_POINT('Ctrl Pts',(-1.0904966249175,2.00135053161119,11.8606756249931));
#76243=CARTESIAN_POINT('Ctrl Pts',(-0.925680523765739,1.51065297779157,
11.8868406034525));
#76244=CARTESIAN_POINT('Ctrl Pts',(-0.553184670058425,1.14947860398362,
11.9130629946836));
#76245=CARTESIAN_POINT('Ctrl Pts',(-0.055415031446615,0.999273750331867,
11.9393416867785));
#76246=CARTESIAN_POINT('Ctrl Pts',(0.456850692462456,1.09447748037705,11.965675683592));
#76247=CARTESIAN_POINT('Ctrl Pts',(0.869118461065415,1.41484540483791,11.9920638498054));
#76248=CARTESIAN_POINT('Ctrl Pts',(1.08879853435095,1.88964775701972,12.0185051663876));
#76249=CARTESIAN_POINT('Ctrl Pts',(1.06599737677219,2.41333580572711,12.0449982756185));
#76250=CARTESIAN_POINT('Ctrl Pts',(0.804891629262968,2.86900603669412,12.0715424339268));
#76251=CARTESIAN_POINT('Ctrl Pts',(0.362923366288464,3.15451545410712,12.0981353818834));
#76252=CARTESIAN_POINT('Ctrl Pts',(-0.161668688010658,3.20541279760317,
12.1247781162622));
#76253=CARTESIAN_POINT('Ctrl Pts',(-0.652085894169137,3.00945265230991,
12.1514642275061));
#76254=CARTESIAN_POINT('Ctrl Pts',(-0.940446471327969,2.67628514499842,
12.1737473845505));
#76255=CARTESIAN_POINT('Ctrl Pts',(-1.06066013461824,2.35191836336405,12.1915846173031));
#76256=CARTESIAN_POINT('Ctrl Pts',(-1.08088861775694,2.18131633339423,12.2005290550795));
#76257=CARTESIAN_POINT('Ctrl Pts',(-1.08084165385376,2.0946891367405,12.2049801218611));
#76258=CARTESIAN_POINT('Ctrl Pts',(0.91153047167304,2.1,9.62353994288304));
#76259=CARTESIAN_POINT('Ctrl Pts',(0.91105364478002,2.17348405122035,9.62732031744799));
#76260=CARTESIAN_POINT('Ctrl Pts',(0.892967745079117,2.31673902258848,9.63483964861492));
#76261=CARTESIAN_POINT('Ctrl Pts',(0.789521176264839,2.58987098214541,9.64989741724387));
#76262=CARTESIAN_POINT('Ctrl Pts',(0.544564452912013,2.86843394076872,9.668658841039));
#76263=CARTESIAN_POINT('Ctrl Pts',(0.130536318539686,3.03042695712525,9.69112807964226));
#76264=CARTESIAN_POINT('Ctrl Pts',(-0.310330783421158,2.98427236214618,
9.71353513800462));
#76265=CARTESIAN_POINT('Ctrl Pts',(-0.680015491769051,2.74157537674839,
9.73588959548194));
#76266=CARTESIAN_POINT('Ctrl Pts',(-0.896499318571394,2.357167057499,9.75818908021112));
#76267=CARTESIAN_POINT('Ctrl Pts',(-0.912376566341135,1.91732632552379,
9.78043662951247));
#76268=CARTESIAN_POINT('Ctrl Pts',(-0.725024155965477,1.52017204573209,
9.80263291027502));
#76269=CARTESIAN_POINT('Ctrl Pts',(-0.377066297404346,1.25391115517105,
9.82477967943719));
#76270=CARTESIAN_POINT('Ctrl Pts',(0.0533471125557414,1.17723280759371,
9.84687824938293));
#76271=CARTESIAN_POINT('Ctrl Pts',(0.470060182466133,1.30637765174259,9.86893017531943));
#76272=CARTESIAN_POINT('Ctrl Pts',(0.78036781679815,1.61178376947083,9.89093697531718));
#76273=CARTESIAN_POINT('Ctrl Pts',(0.915629767908127,2.02466884923936,9.91290023450542));
#76274=CARTESIAN_POINT('Ctrl Pts',(0.846390455638519,2.45290065637925,9.93482156821705));
#76275=CARTESIAN_POINT('Ctrl Pts',(0.58887797324273,2.80063439575845,9.95670251565969));
#76276=CARTESIAN_POINT('Ctrl Pts',(0.157895298284613,3.01298640312374,9.98097182074651));
#76277=CARTESIAN_POINT('Ctrl Pts',(-0.377917255020538,2.95989571059473,
10.0076141443979));
#76278=CARTESIAN_POINT('Ctrl Pts',(-0.813700360743258,2.56591121504782,
10.0366162055263));
#76279=CARTESIAN_POINT('Ctrl Pts',(-0.90933677990633,2.08797029208528,10.0607376094115));
#76280=CARTESIAN_POINT('Ctrl Pts',(-0.806016864557925,1.72706447977729,
10.0800087547882));
#76281=CARTESIAN_POINT('Ctrl Pts',(-0.648638252475412,1.49408849163869,
10.0944489361237));
#76282=CARTESIAN_POINT('Ctrl Pts',(-0.426263420033854,1.32255523282061,
10.1088766557053));
#76283=CARTESIAN_POINT('Ctrl Pts',(-0.073366716764664,1.19694055764828,
10.1280985439345));
#76284=CARTESIAN_POINT('Ctrl Pts',(0.342755481993835,1.25443301936784,10.1488935550027));
#76285=CARTESIAN_POINT('Ctrl Pts',(0.688405486121672,1.52715182432036,10.1712661011271));
#76286=CARTESIAN_POINT('Ctrl Pts',(0.862394009352625,1.86110195503896,10.1904256185386));
#76287=CARTESIAN_POINT('Ctrl Pts',(0.881814193602376,2.20582919186377,10.2079731409895));
#76288=CARTESIAN_POINT('Ctrl Pts',(0.785548217129111,2.5008254907576,10.2239156985126));
#76289=CARTESIAN_POINT('Ctrl Pts',(0.56591941828687,2.80169942910186,10.2430370586467));
#76290=CARTESIAN_POINT('Ctrl Pts',(0.133807769973548,3.01703821882315,10.2669184653035));
#76291=CARTESIAN_POINT('Ctrl Pts',(-0.436917678576326,2.91645318725037,
10.2955546153329));
#76292=CARTESIAN_POINT('Ctrl Pts',(-0.835922416842069,2.4971875235335,10.3241712524374));
#76293=CARTESIAN_POINT('Ctrl Pts',(-0.908007865198345,1.92302512682405,
10.3527740090878));
#76294=CARTESIAN_POINT('Ctrl Pts',(-0.625265349485015,1.41856922050494,
10.3813664070234));
#76295=CARTESIAN_POINT('Ctrl Pts',(-0.0980075253033923,1.18038116079578,
10.4099539128241));
#76296=CARTESIAN_POINT('Ctrl Pts',(0.404142738693815,1.28877534199984,10.4353631479262));
#76297=CARTESIAN_POINT('Ctrl Pts',(0.726402174614211,1.58472143067419,10.4576006853765));
#76298=CARTESIAN_POINT('Ctrl Pts',(0.874385876809216,1.92902833247871,10.4766638408478));
#76299=CARTESIAN_POINT('Ctrl Pts',(0.867435595716759,2.30398797603964,10.4957315864257));
#76300=CARTESIAN_POINT('Ctrl Pts',(0.707054269343606,2.64311684354316,10.5148056321417));
#76301=CARTESIAN_POINT('Ctrl Pts',(0.421116724846305,2.8858766210418,10.5338865299558));
#76302=CARTESIAN_POINT('Ctrl Pts',(0.000306317622067648,3.00793566462754,
10.5561570667423));
#76303=CARTESIAN_POINT('Ctrl Pts',(-0.498728080378487,2.88150683444137,
10.581622031038));
#76304=CARTESIAN_POINT('Ctrl Pts',(-0.866739074640701,2.43287565356016,
10.6103008121439));
#76305=CARTESIAN_POINT('Ctrl Pts',(-0.89567648973,1.85273981720578,10.6390059526166));
#76306=CARTESIAN_POINT('Ctrl Pts',(-0.57458622137938,1.36824600602171,10.6677477437704));
#76307=CARTESIAN_POINT('Ctrl Pts',(-0.0273166520720773,1.16859943191723,
10.6965289270857));
#76308=CARTESIAN_POINT('Ctrl Pts',(0.469506483946871,1.31533648442313,10.7221489581215));
#76309=CARTESIAN_POINT('Ctrl Pts',(0.771641137123773,1.63753656926365,10.7446015563863));
#76310=CARTESIAN_POINT('Ctrl Pts',(0.874414726399044,1.93595303744339,10.7606572590965));
#76311=CARTESIAN_POINT('Ctrl Pts',(0.877323346348476,2.18455153451786,10.7735139397468));
#76312=CARTESIAN_POINT('Ctrl Pts',(0.820424570946683,2.46929223171017,10.7885230217106));
#76313=CARTESIAN_POINT('Ctrl Pts',(0.64164599771704,2.73689268744519,10.8046210998245));
#76314=CARTESIAN_POINT('Ctrl Pts',(0.322885446846539,2.93618132347737,10.8239692642255));
#76315=CARTESIAN_POINT('Ctrl Pts',(-0.00823321698495057,3.00572801835655,
10.8411845128887));
#76316=CARTESIAN_POINT('Ctrl Pts',(-0.380918433916755,2.92340325825145,
10.8605837425962));
#76317=CARTESIAN_POINT('Ctrl Pts',(-0.686732400828136,2.69475762437649,
10.8800100296679));
#76318=CARTESIAN_POINT('Ctrl Pts',(-0.903601656768487,2.30426172271222,
10.9027121258681));
#76319=CARTESIAN_POINT('Ctrl Pts',(-0.891411633732064,1.77884460545719,
10.9287080284181));
#76320=CARTESIAN_POINT('Ctrl Pts',(-0.527555828750873,1.31001811981728,
10.958031197091));
#76321=CARTESIAN_POINT('Ctrl Pts',(0.0447580861818993,1.14848673179254,
10.9874336854073));
#76322=CARTESIAN_POINT('Ctrl Pts',(0.602941681277028,1.35888446381741,11.0169200010601));
#76323=CARTESIAN_POINT('Ctrl Pts',(0.927970988373135,1.86117278345443,11.0464932429883));
#76324=CARTESIAN_POINT('Ctrl Pts',(0.891255966367144,2.45997746423432,11.0761567696705));
#76325=CARTESIAN_POINT('Ctrl Pts',(0.504702358672154,2.92177668715295,11.105914324334));
#76326=CARTESIAN_POINT('Ctrl Pts',(-0.0167793435795264,3.04771529211323,
11.1324507777199));
#76327=CARTESIAN_POINT('Ctrl Pts',(-0.455338690749746,2.91511037606382,
11.1557367370154));
#76328=CARTESIAN_POINT('Ctrl Pts',(-0.752183284487268,2.65723389205797,
11.1757423237457));
#76329=CARTESIAN_POINT('Ctrl Pts',(-0.916841848233799,2.29878925378214,
11.1957925332484));
#76330=CARTESIAN_POINT('Ctrl Pts',(-0.919776969791426,1.90364303364972,
11.2158918338139));
#76331=CARTESIAN_POINT('Ctrl Pts',(-0.759308358911334,1.54129526233824,
11.2360370757184));
#76332=CARTESIAN_POINT('Ctrl Pts',(-0.463475971789943,1.27646148633192,
11.2562322548172));
#76333=CARTESIAN_POINT('Ctrl Pts',(-0.0837713729081205,1.15625183292691,
11.2764761143988));
#76334=CARTESIAN_POINT('Ctrl Pts',(0.312377222380745,1.20332878815849,11.2967717707931));
#76335=CARTESIAN_POINT('Ctrl Pts',(0.712912934890082,1.4433776123106,11.3205098526284));
#76336=CARTESIAN_POINT('Ctrl Pts',(0.977159827924982,1.92592825997509,11.3477225173613));
#76337=CARTESIAN_POINT('Ctrl Pts',(0.892810604480596,2.54223408268594,11.3784572591806));
#76338=CARTESIAN_POINT('Ctrl Pts',(0.457739726643327,2.98944426773445,11.4093130261963));
#76339=CARTESIAN_POINT('Ctrl Pts',(-0.160800171609709,3.09173229952906,
11.4402913214941));
#76340=CARTESIAN_POINT('Ctrl Pts',(-0.720733679185758,2.80499075517892,
11.4713968913498));
#76341=CARTESIAN_POINT('Ctrl Pts',(-1.00281663250133,2.23968124921094,11.5026276832156));
#76342=CARTESIAN_POINT('Ctrl Pts',(-0.89360612273627,1.61492108193344,11.5339875295911));
#76343=CARTESIAN_POINT('Ctrl Pts',(-0.432776176189375,1.17483510359387,
11.5654765787301));
#76344=CARTESIAN_POINT('Ctrl Pts',(0.201746101425125,1.09496619635988,11.5970988524765));
#76345=CARTESIAN_POINT('Ctrl Pts',(0.762475338330419,1.4081509930752,11.6288524812263));
#76346=CARTESIAN_POINT('Ctrl Pts',(1.028668635657,1.9956937457661,11.6607399754007));
#76347=CARTESIAN_POINT('Ctrl Pts',(0.893491389235042,2.62901163607681,11.6927620183401));
#76348=CARTESIAN_POINT('Ctrl Pts',(0.406345553247394,3.06044896638264,11.7249195550277));
#76349=CARTESIAN_POINT('Ctrl Pts',(-0.189814472656564,3.11306137855792,
11.7545217329727));
#76350=CARTESIAN_POINT('Ctrl Pts',(-0.666752905623271,2.87149615924449,
11.7815329051351));
#76351=CARTESIAN_POINT('Ctrl Pts',(-0.949541402730192,2.48086457287139,
11.8059197450728));
#76352=CARTESIAN_POINT('Ctrl Pts',(-1.021591881002,2.00217060603226,11.8303836532157));
#76353=CARTESIAN_POINT('Ctrl Pts',(-0.865475264992205,1.5425140203653,11.8549246178449));
#76354=CARTESIAN_POINT('Ctrl Pts',(-0.514682296535199,1.20465835352623,
11.8795426851172));
#76355=CARTESIAN_POINT('Ctrl Pts',(-0.0465088282181845,1.06508734362675,
11.9042378039794));
#76356=CARTESIAN_POINT('Ctrl Pts',(0.434999468617669,1.15623157178554,11.9290098923686));
#76357=CARTESIAN_POINT('Ctrl Pts',(0.822155795806256,1.45914698732355,11.953858817131));
#76358=CARTESIAN_POINT('Ctrl Pts',(1.02773081257076,1.90734105827644,11.9787843903828));
#76359=CARTESIAN_POINT('Ctrl Pts',(1.00458945105254,2.40139718661437,12.0037864018186));
#76360=CARTESIAN_POINT('Ctrl Pts',(0.756530865593507,2.83103044687003,12.0288645331178));
#76361=CARTESIAN_POINT('Ctrl Pts',(0.337665092123472,3.0996729282449,12.054018544057));
#76362=CARTESIAN_POINT('Ctrl Pts',(-0.159203321446335,3.14628016851133,
12.0792478546339));
#76363=CARTESIAN_POINT('Ctrl Pts',(-0.623545249266301,2.95897818066081,
12.1045524799382));
#76364=CARTESIAN_POINT('Ctrl Pts',(-0.896243240370551,2.64197021732172,
12.1257012707751));
#76365=CARTESIAN_POINT('Ctrl Pts',(-1.0094947193235,2.33329207765941,12.142657782671));
#76366=CARTESIAN_POINT('Ctrl Pts',(-1.02817517058789,2.17121348557861,12.1511526949405));
#76367=CARTESIAN_POINT('Ctrl Pts',(-1.0278656018829,2.08874423191622,12.1553877468729));
#76368=CARTESIAN_POINT('Ctrl Pts',(1.01797127075135,2.1,9.6476237796153));
#76369=CARTESIAN_POINT('Ctrl Pts',(1.01739759936018,2.18170177247089,9.6518273032171));
#76370=CARTESIAN_POINT('Ctrl Pts',(0.997075497366153,2.34197250729824,9.66024085688616));
#76371=CARTESIAN_POINT('Ctrl Pts',(0.881531712257153,2.64643874397719,9.67702980010063));
#76372=CARTESIAN_POINT('Ctrl Pts',(0.607964326124389,2.95729913578499,9.69797635490342));
#76373=CARTESIAN_POINT('Ctrl Pts',(0.146117437660257,3.13759906306215,9.7230321873618));
#76374=CARTESIAN_POINT('Ctrl Pts',(-0.345304308274442,3.08590135078223,
9.74801368543017));
#76375=CARTESIAN_POINT('Ctrl Pts',(-0.756976146008362,2.81525529634975,
9.77291797455823));
#76376=CARTESIAN_POINT('Ctrl Pts',(-0.997717508088822,2.38715531499302,
9.79774602149462));
#76377=CARTESIAN_POINT('Ctrl Pts',(-1.01506151072978,1.89783538729067,9.82249714066535));
#76378=CARTESIAN_POINT('Ctrl Pts',(-0.806515684265896,1.45651892696938,
9.84717145196844));
#76379=CARTESIAN_POINT('Ctrl Pts',(-0.419883171833556,1.16108253062822,
9.87176878241307));
#76380=CARTESIAN_POINT('Ctrl Pts',(0.0577202993719235,1.07634276501048,
9.89628915431694));
#76381=CARTESIAN_POINT('Ctrl Pts',(0.519484551037105,1.21981225012954,9.920732569481));
#76382=CARTESIAN_POINT('Ctrl Pts',(0.862788216351348,1.5581888500835,9.94509910118577));
#76383=CARTESIAN_POINT('Ctrl Pts',(1.01202267624069,2.01488089045114,9.96938887034206));
#76384=CARTESIAN_POINT('Ctrl Pts',(0.935188214037597,2.4877796210854,9.99360202114725));
#76385=CARTESIAN_POINT('Ctrl Pts',(0.650855911768474,2.87110216479637,10.0177388018848));
#76386=CARTESIAN_POINT('Ctrl Pts',(0.175957669185131,3.10461154539347,10.0444727503347));
#76387=CARTESIAN_POINT('Ctrl Pts',(-0.413167711787148,3.04566930798458,
10.0737725308512));
#76388=CARTESIAN_POINT('Ctrl Pts',(-0.890919517513664,2.61284831774276,
10.1056022275272));
#76389=CARTESIAN_POINT('Ctrl Pts',(-0.995095843058391,2.08946109816007,
10.1320154342246));
#76390=CARTESIAN_POINT('Ctrl Pts',(-0.881857808909978,1.69509979853437,
10.1530795785575));
#76391=CARTESIAN_POINT('Ctrl Pts',(-0.709848962015113,1.4408985803547,10.1688450423686));
#76392=CARTESIAN_POINT('Ctrl Pts',(-0.467231119511972,1.2540641047854,10.1845779386659));
#76393=CARTESIAN_POINT('Ctrl Pts',(-0.0828134109998774,1.11758673889094,
10.2055113384881));
#76394=CARTESIAN_POINT('Ctrl Pts',(0.369452164886118,1.18058988554342,10.2281221188686));
#76395=CARTESIAN_POINT('Ctrl Pts',(0.7440178520349,1.47670100636996,10.252386384903));
#76396=CARTESIAN_POINT('Ctrl Pts',(0.932024497398691,1.83837824126288,10.2731281089248));
#76397=CARTESIAN_POINT('Ctrl Pts',(0.952644215160796,2.21088284443421,10.2920911026948));
#76398=CARTESIAN_POINT('Ctrl Pts',(0.848525607611788,2.52898866039414,10.3092894684908));
#76399=CARTESIAN_POINT('Ctrl Pts',(0.611667175977124,2.85284466806143,10.3298862729762));
#76400=CARTESIAN_POINT('Ctrl Pts',(0.146965686342124,3.08368825181904,10.3555582533163));
#76401=CARTESIAN_POINT('Ctrl Pts',(-0.464353171151464,2.975108638042,10.386243371414));
#76402=CARTESIAN_POINT('Ctrl Pts',(-0.889867125642017,2.52677225013601,
10.416811145006));
#76403=CARTESIAN_POINT('Ctrl Pts',(-0.965740853436312,1.91549196386248,
10.4472632931353));
#76404=CARTESIAN_POINT('Ctrl Pts',(-0.665009451066436,1.3807587525135,10.4776028117676));
#76405=CARTESIAN_POINT('Ctrl Pts',(-0.107204061616131,1.12977374293364,
10.5078318049331));
#76406=CARTESIAN_POINT('Ctrl Pts',(0.42164025457547,1.24476928475959,10.534607434734));
#76407=CARTESIAN_POINT('Ctrl Pts',(0.759718865620174,1.55601522514066,10.5579665142426));
#76408=CARTESIAN_POINT('Ctrl Pts',(0.914324817649136,1.91696166575999,10.5779435538898));
#76409=CARTESIAN_POINT('Ctrl Pts',(0.906569512809831,2.3088532786035,10.5978754983735));
#76410=CARTESIAN_POINT('Ctrl Pts',(0.738905867542777,2.6621948935939,10.6177631360867));
#76411=CARTESIAN_POINT('Ctrl Pts',(0.441235879468831,2.91426160241039,10.637607949746));
#76412=CARTESIAN_POINT('Ctrl Pts',(0.00456059090871799,3.04028767733564,
10.6607115176031));
#76413=CARTESIAN_POINT('Ctrl Pts',(-0.511236862099568,2.90870901173369,
10.6870502515913));
#76414=CARTESIAN_POINT('Ctrl Pts',(-0.889437964423829,2.44600479875113,
10.7165883937909));
#76415=CARTESIAN_POINT('Ctrl Pts',(-0.918086783201766,1.85081981438801,
10.7460453215445));
#76416=CARTESIAN_POINT('Ctrl Pts',(-0.589115930172112,1.35637751165594,
10.7754190974754));
#76417=CARTESIAN_POINT('Ctrl Pts',(-0.0318173159979765,1.15422575921844,
10.8047148729315));
#76418=CARTESIAN_POINT('Ctrl Pts',(0.471469629709559,1.30389074576235,10.8306915854604));
#76419=CARTESIAN_POINT('Ctrl Pts',(0.776137002363046,1.62977906851438,10.8533714866067));
#76420=CARTESIAN_POINT('Ctrl Pts',(0.879201460171853,1.93054705157793,10.8695469973497));
#76421=CARTESIAN_POINT('Ctrl Pts',(0.881792886165801,2.1804515005481,10.8824726714454));
#76422=CARTESIAN_POINT('Ctrl Pts',(0.824281002588274,2.46622964067337,10.8975414512373));
#76423=CARTESIAN_POINT('Ctrl Pts',(0.644771590343777,2.73390655574528,10.9136676846433));
#76424=CARTESIAN_POINT('Ctrl Pts',(0.326172155862462,2.93244834317385,10.932988933727));
#76425=CARTESIAN_POINT('Ctrl Pts',(-0.00389180032462818,3.00123878482214,
10.9501482361413));
#76426=CARTESIAN_POINT('Ctrl Pts',(-0.374069531768034,2.91882600059989,
10.9694246322533));
#76427=CARTESIAN_POINT('Ctrl Pts',(-0.676770714493534,2.69175674503232,
10.9886811485452));
#76428=CARTESIAN_POINT('Ctrl Pts',(-0.890457839169829,2.30547459389054,
11.0111195762753));
#76429=CARTESIAN_POINT('Ctrl Pts',(-0.877420955696323,1.78796824742822,
11.0367326718632));
#76430=CARTESIAN_POINT('Ctrl Pts',(-0.519542383046932,1.32879774668238,
11.0655040102286));
#76431=CARTESIAN_POINT('Ctrl Pts',(0.0399490643477976,1.17212920136542,
11.0942383879097));
#76432=CARTESIAN_POINT('Ctrl Pts',(0.582718196329541,1.37801627095207,11.1229395555505));
#76433=CARTESIAN_POINT('Ctrl Pts',(0.896745247812362,1.86556201558046,11.1516121597076));
#76434=CARTESIAN_POINT('Ctrl Pts',(0.860059296447071,2.44367223802959,11.1802608561107));
#76435=CARTESIAN_POINT('Ctrl Pts',(0.487287812128845,2.88705936152277,11.2088896613278));
#76436=CARTESIAN_POINT('Ctrl Pts',(-0.0126793677166393,3.00666626742902,
11.2343251238526));
#76437=CARTESIAN_POINT('Ctrl Pts',(-0.431368788585849,2.8792260766813,11.256572216763));
#76438=CARTESIAN_POINT('Ctrl Pts',(-0.713776887062524,2.63297361864757,
11.2756367991276));
#76439=CARTESIAN_POINT('Ctrl Pts',(-0.869675700701866,2.29192787722306,
11.2947015047042));
#76440=CARTESIAN_POINT('Ctrl Pts',(-0.871754349920706,1.91719764545345,
11.3137629349912));
#76441=CARTESIAN_POINT('Ctrl Pts',(-0.719284033324151,1.57464106746168,
11.3328277507209));
#76442=CARTESIAN_POINT('Ctrl Pts',(-0.439566572325031,1.32517731125754,
11.3518929564459));
#76443=CARTESIAN_POINT('Ctrl Pts',(-0.0817424075530357,1.21263403993146,
11.3709626858035));
#76444=CARTESIAN_POINT('Ctrl Pts',(0.290412185317624,1.25756731850338,11.3900351084129));
#76445=CARTESIAN_POINT('Ctrl Pts',(0.6655187140127,1.48335758138164,11.4122929276818));
#76446=CARTESIAN_POINT('Ctrl Pts',(0.911646236291874,1.93514475264904,11.4377467160272));
#76447=CARTESIAN_POINT('Ctrl Pts',(0.831748897734901,2.5094592535539,11.4664011327166));
#76448=CARTESIAN_POINT('Ctrl Pts',(0.42653080354753,2.92417639523713,11.4950808407273));
#76449=CARTESIAN_POINT('Ctrl Pts',(-0.14681541068467,3.01769219474351,11.5237915175372));
#76450=CARTESIAN_POINT('Ctrl Pts',(-0.663565009681244,2.75164209798711,
11.5525329012227));
#76451=CARTESIAN_POINT('Ctrl Pts',(-0.922343659292911,2.23017004462751,
11.5813153753167));
#76452=CARTESIAN_POINT('Ctrl Pts',(-0.82072898896079,1.65621568500738,11.6101398171542));
#76453=CARTESIAN_POINT('Ctrl Pts',(-0.397384311892478,1.25368822232143,
11.6390127119604));
#76454=CARTESIAN_POINT('Ctrl Pts',(0.183049465176804,1.18189553873558,11.6679338789258));
#76455=CARTESIAN_POINT('Ctrl Pts',(0.694090218061655,1.46877497685727,11.6969126968832));
#76456=CARTESIAN_POINT('Ctrl Pts',(0.935321267131387,2.00426367937146,11.725950863301));
#76457=CARTESIAN_POINT('Ctrl Pts',(0.811264797020236,2.57949055623937,11.7550527002716));
#76458=CARTESIAN_POINT('Ctrl Pts',(0.368614734530845,2.96985351560571,11.7842218445857));
#76459=CARTESIAN_POINT('Ctrl Pts',(-0.171225999656093,3.01635946820556,
11.8110263031446));
#76460=CARTESIAN_POINT('Ctrl Pts',(-0.601966326773585,2.79712243250774,
11.8354476933365));
#76461=CARTESIAN_POINT('Ctrl Pts',(-0.856635786021019,2.44387729840415,
11.8574712161541));
#76462=CARTESIAN_POINT('Ctrl Pts',(-0.920780349043476,2.01195470589779,
11.8795401240644));
#76463=CARTESIAN_POINT('Ctrl Pts',(-0.779294306257107,1.59802697812281,
11.901656095375));
#76464=CARTESIAN_POINT('Ctrl Pts',(-0.462897586535699,1.29448147638559,
11.9238205287533));
#76465=CARTESIAN_POINT('Ctrl Pts',(-0.0415426238937191,1.1697542653126,
11.9460349558951));
#76466=CARTESIAN_POINT('Ctrl Pts',(0.391061638465007,1.25250459967951,11.968300755167));
#76467=CARTESIAN_POINT('Ctrl Pts',(0.738250016927639,1.52522229421188,11.9906194062099));
#76468=CARTESIAN_POINT('Ctrl Pts',(0.921992585201663,1.92784239197626,12.012992073041));
#76469=CARTESIAN_POINT('Ctrl Pts',(0.900393282784436,2.37097208359455,12.0354205108322));
#76470=CARTESIAN_POINT('Ctrl Pts',(0.677271806505565,2.75575131201869,12.0579050641389));
#76471=CARTESIAN_POINT('Ctrl Pts',(0.301444205308227,2.99578096804062,12.0804491519056));
#76472=CARTESIAN_POINT('Ctrl Pts',(-0.143737457268676,3.03675145400947,
12.1030492099952));
#76473=CARTESIAN_POINT('Ctrl Pts',(-0.559307355611989,2.86815774679212,
12.1257171734423));
#76474=CARTESIAN_POINT('Ctrl Pts',(-0.802911717332437,2.58405107780456,
12.1446443351558));
#76475=CARTESIAN_POINT('Ctrl Pts',(-0.903878021992128,2.30723336901298,
12.159841505477));
#76476=CARTESIAN_POINT('Ctrl Pts',(-0.920298150261432,2.16243836817539,
12.1674290389266));
#76477=CARTESIAN_POINT('Ctrl Pts',(-0.919891595085131,2.08831921315703,
12.1712341381108));
#76478=CARTESIAN_POINT('Ctrl Pts',(1.10362653322406,2.1,9.57968132589776));
#76479=CARTESIAN_POINT('Ctrl Pts',(1.10332385859517,2.18836737691272,9.58422494608045));
#76480=CARTESIAN_POINT('Ctrl Pts',(1.08191344062549,2.3625059514978,9.59336230827583));
#76481=CARTESIAN_POINT('Ctrl Pts',(0.957835600463251,2.69310587840379,9.61156968419157));
#76482=CARTESIAN_POINT('Ctrl Pts',(0.661841991943411,3.03223916038163,9.63434167170328));
#76483=CARTESIAN_POINT('Ctrl Pts',(0.159943307176907,3.23039051797218,9.66161187516289));
#76484=CARTESIAN_POINT('Ctrl Pts',(-0.376051688795035,3.17620291801981,
9.68885171355759));
#76485=CARTESIAN_POINT('Ctrl Pts',(-0.826750739733302,2.88245239593225,
9.71604756503803));
#76486=CARTESIAN_POINT('Ctrl Pts',(-1.09190901430628,2.41533590672408,9.74320319226711));
#76487=CARTESIAN_POINT('Ctrl Pts',(-1.11305483350507,1.87947767032364,9.77031460500698));
#76488=CARTESIAN_POINT('Ctrl Pts',(-0.88625766736864,1.39450346688661,9.79738131769857));
#76489=CARTESIAN_POINT('Ctrl Pts',(-0.462890049527857,1.06828884415501,
9.82440133351827));
#76490=CARTESIAN_POINT('Ctrl Pts',(0.0620431770221235,0.972966819483573,
9.85137337108375));
#76491=CARTESIAN_POINT('Ctrl Pts',(0.571236025368607,1.12891854941223,9.87829586868765));
#76492=CARTESIAN_POINT('Ctrl Pts',(0.951314593883381,1.50051940417938,9.9051673999022));
#76493=CARTESIAN_POINT('Ctrl Pts',(1.11812369875706,2.0040613394318,9.93198652208759));
#76494=CARTESIAN_POINT('Ctrl Pts',(1.03532433897197,2.52711479570303,9.95875180884655));
#76495=CARTESIAN_POINT('Ctrl Pts',(0.722426325350036,2.95256083044233,9.9854620047878));
#76496=CARTESIAN_POINT('Ctrl Pts',(0.197440843038474,3.21337088955047,10.0150770435447));
#76497=CARTESIAN_POINT('Ctrl Pts',(-0.456162767182428,3.15073737091323,
10.047572536222));
#76498=CARTESIAN_POINT('Ctrl Pts',(-0.988651479746515,2.67238263836449,
10.0829168835724));
#76499=CARTESIAN_POINT('Ctrl Pts',(-1.10688911431785,2.09107215671169,10.1122789590279));
#76500=CARTESIAN_POINT('Ctrl Pts',(-0.982706695062194,1.65185618948298,
10.1357121466742));
#76501=CARTESIAN_POINT('Ctrl Pts',(-0.792422518102662,1.3681585717153,10.1532592369429));
#76502=CARTESIAN_POINT('Ctrl Pts',(-0.523124675612585,1.15901941614237,
10.1707779412534));
#76503=CARTESIAN_POINT('Ctrl Pts',(-0.0955313023476177,1.0052357524766,
10.1940973000699));
#76504=CARTESIAN_POINT('Ctrl Pts',(0.408862852638258,1.07334669481587,10.2193005196674));
#76505=CARTESIAN_POINT('Ctrl Pts',(0.827965416044339,1.40185468333059,10.2463619074908));
#76506=CARTESIAN_POINT('Ctrl Pts',(1.03939646109892,1.80450850302264,10.2695041218372));
#76507=CARTESIAN_POINT('Ctrl Pts',(1.06413743020716,2.22016319496911,10.2906690517014));
#76508=CARTESIAN_POINT('Ctrl Pts',(0.949371402568083,2.57577634655705,10.3098696021912));
#76509=CARTESIAN_POINT('Ctrl Pts',(0.68639441872527,2.93849673521478,10.3328687806801));
#76510=CARTESIAN_POINT('Ctrl Pts',(0.168455748548128,3.19850041638645,10.3615416008252));
#76511=CARTESIAN_POINT('Ctrl Pts',(-0.514981141538362,3.08006574061132,
10.395821174426));
#76512=CARTESIAN_POINT('Ctrl Pts',(-0.992484975124322,2.58115298612403,
10.4299727529598));
#76513=CARTESIAN_POINT('Ctrl Pts',(-1.08011179202778,1.89857319405739,10.4639941490101));
#76514=CARTESIAN_POINT('Ctrl Pts',(-0.746677452129509,1.2998396969781,10.4978844286978));
#76515=CARTESIAN_POINT('Ctrl Pts',(-0.124919825186299,1.01695088669628,
10.5316419697814));
#76516=CARTESIAN_POINT('Ctrl Pts',(0.465959941776284,1.14285421449709,10.5615302638894));
#76517=CARTESIAN_POINT('Ctrl Pts',(0.84465605145784,1.48855843425709,10.587594536741));
#76518=CARTESIAN_POINT('Ctrl Pts',(1.0187956561827,1.8904143255726,10.6098754554049));
#76519=CARTESIAN_POINT('Ctrl Pts',(1.01199111001941,2.3273475800656,10.6320960171808));
#76520=CARTESIAN_POINT('Ctrl Pts',(0.826831590311268,2.72185411327491,10.6542558772749));
#76521=CARTESIAN_POINT('Ctrl Pts',(0.496525135839689,3.00395863731658,10.6763551851293));
#76522=CARTESIAN_POINT('Ctrl Pts',(0.0111327324295966,3.14626897049278,
10.7020667852219));
#76523=CARTESIAN_POINT('Ctrl Pts',(-0.562996470319803,3.00232707281753,
10.7313506493589));
#76524=CARTESIAN_POINT('Ctrl Pts',(-0.985170581520541,2.49014805337043,
10.7641569125056));
#76525=CARTESIAN_POINT('Ctrl Pts',(-1.01964968628344,1.83010686065805,10.796826521172));
#76526=CARTESIAN_POINT('Ctrl Pts',(-0.657524636731054,1.2809574776055,10.82935855228));
#76527=CARTESIAN_POINT('Ctrl Pts',(-0.0421227513948548,1.05489108814208,
10.8617537289328));
#76528=CARTESIAN_POINT('Ctrl Pts',(0.514174199288179,1.21785062909781,10.8904278519412));
#76529=CARTESIAN_POINT('Ctrl Pts',(0.85154389222315,1.57569141984744,10.9154296374838));
#76530=CARTESIAN_POINT('Ctrl Pts',(0.966417014836512,1.90635215236884,10.9332377402664));
#76531=CARTESIAN_POINT('Ctrl Pts',(0.970453646751313,2.18120687331145,10.9474542331084));
#76532=CARTESIAN_POINT('Ctrl Pts',(0.90859469374289,2.4956012577166,10.9640168231539));
#76533=CARTESIAN_POINT('Ctrl Pts',(0.712752704384257,2.79023506214752,10.9817165375888));
#76534=CARTESIAN_POINT('Ctrl Pts',(0.364433695189235,3.00937789540993,11.002897218119));
#76535=CARTESIAN_POINT('Ctrl Pts',(0.0034024942377313,3.08620224921852,
11.0216801159058));
#76536=CARTESIAN_POINT('Ctrl Pts',(-0.401645366979633,2.99780965747371,
11.0427525334315));
#76537=CARTESIAN_POINT('Ctrl Pts',(-0.733040599057254,2.75137242952113,
11.0637659149067));
#76538=CARTESIAN_POINT('Ctrl Pts',(-0.967642155109252,2.33143421543358,
11.0882140885227));
#76539=CARTESIAN_POINT('Ctrl Pts',(-0.955682954326625,1.76869539969966,
11.1160579226578));
#76540=CARTESIAN_POINT('Ctrl Pts',(-0.569539517922979,1.26924071592032,
11.1472543095408));
#76541=CARTESIAN_POINT('Ctrl Pts',(0.0348519939173318,1.09745482173835,
11.1783238828312));
#76542=CARTESIAN_POINT('Ctrl Pts',(0.62100013835726,1.31719642390597,11.2092686904388));
#76543=CARTESIAN_POINT('Ctrl Pts',(0.96064358272864,1.84006069348993,11.2400905755795));
#76544=CARTESIAN_POINT('Ctrl Pts',(0.923712874736882,2.45983807259137,11.2707915176385));
#76545=CARTESIAN_POINT('Ctrl Pts',(0.527253109689211,2.93507386065005,11.3013740167069));
#76546=CARTESIAN_POINT('Ctrl Pts',(-0.00465921901833066,3.06447451657243,
11.3284545295349));
#76547=CARTESIAN_POINT('Ctrl Pts',(-0.449822784075272,2.93095416511392,
11.3520772589442));
#76548=CARTESIAN_POINT('Ctrl Pts',(-0.750117905009269,2.67126179915912,
11.3722760149046));
#76549=CARTESIAN_POINT('Ctrl Pts',(-0.916368328645713,2.31143790952571,
11.3924246439911));
#76550=CARTESIAN_POINT('Ctrl Pts',(-0.920169991093076,1.91625186699829,
11.4125264404411));
#76551=CARTESIAN_POINT('Ctrl Pts',(-0.761222390223333,1.55523216818356,
11.4325793615504));
#76552=CARTESIAN_POINT('Ctrl Pts',(-0.468713235571315,1.29223530601167,
11.4525866575616));
#76553=CARTESIAN_POINT('Ctrl Pts',(-0.0945728793433094,1.17291557007476,
11.4725475641567));
#76554=CARTESIAN_POINT('Ctrl Pts',(0.294277762638305,1.21828642696366,11.4924650411748));
#76555=CARTESIAN_POINT('Ctrl Pts',(0.686000429294125,1.45195139999478,11.515651150288));
#76556=CARTESIAN_POINT('Ctrl Pts',(0.943285829534123,1.92015599730346,11.5420752789794));
#76557=CARTESIAN_POINT('Ctrl Pts',(0.862784257153681,2.51453311516829,11.5717107622048));
#76558=CARTESIAN_POINT('Ctrl Pts',(0.446786716728484,2.94334169871474,11.6012565534465));
#76559=CARTESIAN_POINT('Ctrl Pts',(-0.141294894410705,3.04141484108333,
11.6307150656786));
#76560=CARTESIAN_POINT('Ctrl Pts',(-0.670496611937673,2.7713159237941,11.6600938870429));
#76561=CARTESIAN_POINT('Ctrl Pts',(-0.935835849607687,2.24134218677815,
11.6893911557916));
#76562=CARTESIAN_POINT('Ctrl Pts',(-0.834835581082013,1.65900363230969,
11.7186141015149));
#76563=CARTESIAN_POINT('Ctrl Pts',(-0.408739935114945,1.25103259511225,
11.7477640283533));
#76564=CARTESIAN_POINT('Ctrl Pts',(0.17478220598524,1.17681438957091,11.7768498186601));
#76565=CARTESIAN_POINT('Ctrl Pts',(0.687633529056747,1.46239191516575,11.8058695158234));
#76566=CARTESIAN_POINT('Ctrl Pts',(0.930087435743391,1.99572519490728,11.8348301864855));
#76567=CARTESIAN_POINT('Ctrl Pts',(0.808788711597153,2.56759105376501,11.8637352173148));
#76568=CARTESIAN_POINT('Ctrl Pts',(0.372142364372509,2.95527860777237,11.8925892923752));
#76569=CARTESIAN_POINT('Ctrl Pts',(-0.159618674117736,3.00289391958003,
11.9189950219207));
#76570=CARTESIAN_POINT('Ctrl Pts',(-0.583320569409584,2.78916288240356,
11.94297075703));
#76571=CARTESIAN_POINT('Ctrl Pts',(-0.833868275993026,2.44427205908894,
11.9645263067009));
#76572=CARTESIAN_POINT('Ctrl Pts',(-0.897983936371958,2.02295745107859,
11.9860615833256));
#76573=CARTESIAN_POINT('Ctrl Pts',(-0.761752582443683,1.61969407972814,
12.0075782437171));
#76574=CARTESIAN_POINT('Ctrl Pts',(-0.455842358238346,1.32411057372178,
12.0290782429238));
#76575=CARTESIAN_POINT('Ctrl Pts',(-0.048683049811289,1.20201416224315,
12.0505634713502));
#76576=CARTESIAN_POINT('Ctrl Pts',(0.36885285869097,1.28035488007001,12.0720357864435));
#76577=CARTESIAN_POINT('Ctrl Pts',(0.703682538373774,1.54146396668747,12.0934971695462));
#76578=CARTESIAN_POINT('Ctrl Pts',(0.881249234813493,1.92696228266429,12.1149492451026));
#76579=CARTESIAN_POINT('Ctrl Pts',(0.862077846834763,2.35080266214842,12.1363944669441));
#76580=CARTESIAN_POINT('Ctrl Pts',(0.650581145027489,2.71849457060569,12.1578334355429));
#76581=CARTESIAN_POINT('Ctrl Pts',(0.293950474197431,2.94800565088334,12.179270942516));
#76582=CARTESIAN_POINT('Ctrl Pts',(-0.12814443883228,2.98834258470624,12.2007023996387));
#76583=CARTESIAN_POINT('Ctrl Pts',(-0.521799371244013,2.83016779854685,
12.222144175476));
#76584=CARTESIAN_POINT('Ctrl Pts',(-0.752511019951562,2.562980435684,12.2399948578996));
#76585=CARTESIAN_POINT('Ctrl Pts',(-0.848550148047341,2.30251473117147,
12.2543110264422));
#76586=CARTESIAN_POINT('Ctrl Pts',(-0.864472773112078,2.16656466527785,
12.2614376415572));
#76587=CARTESIAN_POINT('Ctrl Pts',(-0.864339839017289,2.09666417179271,
12.2650284080295));
#76588=CARTESIAN_POINT('Ctrl Pts',(1.10329394384097,2.1,9.47044698901065));
#76589=CARTESIAN_POINT('Ctrl Pts',(1.10342577318052,2.18844051481166,9.47499047623415));
#76590=CARTESIAN_POINT('Ctrl Pts',(1.08292697012135,2.36279317326597,9.48413095460293));
#76591=CARTESIAN_POINT('Ctrl Pts',(0.960358942581555,2.69455029900241,9.50236886786829));
#76592=CARTESIAN_POINT('Ctrl Pts',(0.665197290461623,3.03649933706296,9.52521501416534));
#76593=CARTESIAN_POINT('Ctrl Pts',(0.161391500207772,3.23853294280124,9.55264408464405));
#76594=CARTESIAN_POINT('Ctrl Pts',(-0.3793961911153,3.18679347595313,9.58010840950997));
#76595=CARTESIAN_POINT('Ctrl Pts',(-0.836587092669218,2.89228198671027,
9.60759595890492));
#76596=CARTESIAN_POINT('Ctrl Pts',(-1.10781716561319,2.42036554420295,9.63510948939038));
#76597=CARTESIAN_POINT('Ctrl Pts',(-1.13221150762356,1.87614146775605,9.66264511777613));
#76598=CARTESIAN_POINT('Ctrl Pts',(-0.903913086637555,1.38105914971141,
9.69020192194118));
#76599=CARTESIAN_POINT('Ctrl Pts',(-0.473548122300964,1.04575615380141,
9.717777663979));
#76600=CARTESIAN_POINT('Ctrl Pts',(0.0630410671544533,0.945336835228206,
9.74537069120911));
#76601=CARTESIAN_POINT('Ctrl Pts',(0.586155308009602,1.10248110373778,9.77297906556861));
#76602=CARTESIAN_POINT('Ctrl Pts',(0.97896721945666,1.48242126689961,9.80060095834541));
#76603=CARTESIAN_POINT('Ctrl Pts',(1.15366073282743,2.00041306644017,9.82823441377605));
#76604=CARTESIAN_POINT('Ctrl Pts',(1.07104056272652,2.54117175963957,9.85587763787474));
#76605=CARTESIAN_POINT('Ctrl Pts',(0.749438508422974,2.98341757445515,9.88352858181668));
#76606=CARTESIAN_POINT('Ctrl Pts',(0.206071066343861,3.25703059287624,9.91425882120625));
#76607=CARTESIAN_POINT('Ctrl Pts',(-0.474407586679752,3.19565870375735,
9.94806588138852));
#76608=CARTESIAN_POINT('Ctrl Pts',(-1.03300889611883,2.69951233227857,9.9849483264369));
#76609=CARTESIAN_POINT('Ctrl Pts',(-1.16019631587872,2.09158946634905,10.0156839772865));
#76610=CARTESIAN_POINT('Ctrl Pts',(-1.03231832446509,1.63001844177956,10.0402706670585));
#76611=CARTESIAN_POINT('Ctrl Pts',(-0.833926194436441,1.3308462035937,10.0587080269736));
#76612=CARTESIAN_POINT('Ctrl Pts',(-0.551677262472857,1.10925403577857,
10.0771425266126));
#76613=CARTESIAN_POINT('Ctrl Pts',(-0.10187955485641,0.944796612224074,
10.101718548257));
#76614=CARTESIAN_POINT('Ctrl Pts',(0.431214416355967,1.01375057212635,10.1283277734834));
#76615=CARTESIAN_POINT('Ctrl Pts',(0.876826776842245,1.35918124772021,10.1569777420977));
#76616=CARTESIAN_POINT('Ctrl Pts',(1.10339080843243,1.78510336459368,10.1815245804526));
#76617=CARTESIAN_POINT('Ctrl Pts',(1.13206152107633,2.22668002384982,10.2040138041529));
#76618=CARTESIAN_POINT('Ctrl Pts',(1.01189652022592,2.60586469879454,10.2244501669362));
#76619=CARTESIAN_POINT('Ctrl Pts',(0.733641827560973,2.99397501004058,10.2489638393176));
#76620=CARTESIAN_POINT('Ctrl Pts',(0.182030027737687,3.27476674135432,10.2795811045697));
#76621=CARTESIAN_POINT('Ctrl Pts',(-0.550583503416367,3.15205884217581,
10.3162865257328));
#76622=CARTESIAN_POINT('Ctrl Pts',(-1.06629714487458,2.61925513593017,10.3529493854541));
#76623=CARTESIAN_POINT('Ctrl Pts',(-1.16476552168883,1.88502805076137,10.389566510702));
#76624=CARTESIAN_POINT('Ctrl Pts',(-0.808598434657076,1.23689007105085,
10.4261328995388));
#76625=CARTESIAN_POINT('Ctrl Pts',(-0.137754182673855,0.927075763803486,
10.4626450549438));
#76626=CARTESIAN_POINT('Ctrl Pts',(0.503690057736241,1.05996953035151,10.495046832965));
#76627=CARTESIAN_POINT('Ctrl Pts',(0.917146925299477,1.4332859468041,10.5233599744073));
#76628=CARTESIAN_POINT('Ctrl Pts',(1.10898999507462,1.86945446726646,10.547598536504));
#76629=CARTESIAN_POINT('Ctrl Pts',(1.10417701875731,2.34555607374905,10.5718072285612));
#76630=CARTESIAN_POINT('Ctrl Pts',(0.904506920874453,2.77711621170411,10.5959851258615));
#76631=CARTESIAN_POINT('Ctrl Pts',(0.545286687123858,3.08732878341821,10.6201303114132));
#76632=CARTESIAN_POINT('Ctrl Pts',(0.015076277217216,3.24595196324875,10.6482602553399));
#76633=CARTESIAN_POINT('Ctrl Pts',(-0.614985359098582,3.09176141069313,
10.6803476073743));
#76634=CARTESIAN_POINT('Ctrl Pts',(-1.08173166535535,2.53202576584709,10.7163683911006));
#76635=CARTESIAN_POINT('Ctrl Pts',(-1.12377096357778,1.80620962017753,10.7522995324198));
#76636=CARTESIAN_POINT('Ctrl Pts',(-0.728194421216213,1.19884669077671,
10.7881432926498));
#76637=CARTESIAN_POINT('Ctrl Pts',(-0.0504048859193792,0.945479795171635,
10.823894484474));
#76638=CARTESIAN_POINT('Ctrl Pts',(0.565533637893201,1.12211398585112,10.8555867339139));
#76639=CARTESIAN_POINT('Ctrl Pts',(0.941120756083501,1.51607388859285,10.8832566231257));
#76640=CARTESIAN_POINT('Ctrl Pts',(1.07041286826489,1.88164852196315,10.9029829474289));
#76641=CARTESIAN_POINT('Ctrl Pts',(1.07656705582405,2.18629511203114,10.918741283468));
#76642=CARTESIAN_POINT('Ctrl Pts',(1.0098967166809,2.53531809348986,10.9371081667145));
#76643=CARTESIAN_POINT('Ctrl Pts',(0.794402553909074,2.86352027212041,10.9567496467229));
#76644=CARTESIAN_POINT('Ctrl Pts',(0.40889178297773,3.10906836029478,10.9802745270439));
#76645=CARTESIAN_POINT('Ctrl Pts',(0.00815355763257491,3.19668782334102,
11.001147248245));
#76646=CARTESIAN_POINT('Ctrl Pts',(-0.442857467235114,3.10091996763833,
11.0245823977996));
#76647=CARTESIAN_POINT('Ctrl Pts',(-0.813178211939382,2.8287505972283,11.0479657008531));
#76648=CARTESIAN_POINT('Ctrl Pts',(-1.0770401110669,2.36262856096914,11.0751885334277));
#76649=CARTESIAN_POINT('Ctrl Pts',(-1.06728995829791,1.73552287386719,11.1062128575312));
#76650=CARTESIAN_POINT('Ctrl Pts',(-0.63990437237774,1.17614522551949,11.1409983119522));
#76651=CARTESIAN_POINT('Ctrl Pts',(0.0333343650464638,0.980625242717132,
11.1756633724409));
#76652=CARTESIAN_POINT('Ctrl Pts',(0.689032879068862,1.2221713856248,11.2102063445392));
#76653=CARTESIAN_POINT('Ctrl Pts',(1.07164646520174,1.80387086382317,11.2446250685247));
#76654=CARTESIAN_POINT('Ctrl Pts',(1.03435973521343,2.49637056796218,11.2789176920495));
#76655=CARTESIAN_POINT('Ctrl Pts',(0.594514117701379,3.02979345316445,11.3130826051129));
#76656=CARTESIAN_POINT('Ctrl Pts',(0.00113517293498442,3.17775143047368,
11.3433361512686));
#76657=CARTESIAN_POINT('Ctrl Pts',(-0.496970892975936,3.0314653783563,11.3697238228033));
#76658=CARTESIAN_POINT('Ctrl Pts',(-0.83402502340684,2.74335862335544,11.3922835866429));
#76659=CARTESIAN_POINT('Ctrl Pts',(-1.02198410458089,2.34262871620902,11.4147839634241));
#76660=CARTESIAN_POINT('Ctrl Pts',(-1.02877477377512,1.90148026772762,11.4372257172929));
#76661=CARTESIAN_POINT('Ctrl Pts',(-0.853709064146416,1.4975378686245,11.4596074513842));
#76662=CARTESIAN_POINT('Ctrl Pts',(-0.529071349327787,1.20223601985623,
11.4819297012752));
#76663=CARTESIAN_POINT('Ctrl Pts',(-0.11260310159066,1.06675150648581,11.5041917957278));
#76664=CARTESIAN_POINT('Ctrl Pts',(0.321122066438537,1.1148034009953,11.5263938697568));
#76665=CARTESIAN_POINT('Ctrl Pts',(0.759040101660253,1.37258360382036,11.5522258911492));
#76666=CARTESIAN_POINT('Ctrl Pts',(1.04846654712675,1.8921835768978,11.58164708954));
#76667=CARTESIAN_POINT('Ctrl Pts',(0.962728469055807,2.55372914824236,11.614609496841));
#76668=CARTESIAN_POINT('Ctrl Pts',(0.503342729250649,3.03274480310301,11.6474349234281));
#76669=CARTESIAN_POINT('Ctrl Pts',(-0.148505353019908,3.1452972651178,11.6801237007564));
#76670=CARTESIAN_POINT('Ctrl Pts',(-0.736533824900539,2.84942649920226,
11.7126750368427));
#76671=CARTESIAN_POINT('Ctrl Pts',(-1.03342940126492,2.26482068051217,11.745090293276));
#76672=CARTESIAN_POINT('Ctrl Pts',(-0.925579138077888,1.62102516068567,
11.7773689257223));
#76673=CARTESIAN_POINT('Ctrl Pts',(-0.458390819496423,1.16854747640426,
11.8095122649012));
#76674=CARTESIAN_POINT('Ctrl Pts',(0.183210697649094,1.08318585175787,11.8415193363785));
#76675=CARTESIAN_POINT('Ctrl Pts',(0.748201733912437,1.39356481279695,11.873392966908));
#76676=CARTESIAN_POINT('Ctrl Pts',(1.01723547526947,1.97645989455456,11.9051330348159));
#76677=CARTESIAN_POINT('Ctrl Pts',(0.888207762276212,2.60244725135778,11.9367408674874));
#76678=CARTESIAN_POINT('Ctrl Pts',(0.414384154620261,3.02802732512881,11.9682174550523));
#76679=CARTESIAN_POINT('Ctrl Pts',(-0.163856583091941,3.08315384425318,
11.9969524799254));
#76680=CARTESIAN_POINT('Ctrl Pts',(-0.625132545752562,2.8538826750464,12.0229809361921));
#76681=CARTESIAN_POINT('Ctrl Pts',(-0.898760814954354,2.48188517101083,
12.0463353731295));
#76682=CARTESIAN_POINT('Ctrl Pts',(-0.970771244314516,2.02685423369152,
12.0696190747675));
#76683=CARTESIAN_POINT('Ctrl Pts',(-0.826406949387474,1.59098975034858,
12.0928329249704));
#76684=CARTESIAN_POINT('Ctrl Pts',(-0.499049475939726,1.2708959531523,12.1159776792298));
#76685=CARTESIAN_POINT('Ctrl Pts',(-0.0626016196059707,1.13717969866151,
12.1390542406761));
#76686=CARTESIAN_POINT('Ctrl Pts',(0.385226093706194,1.21844555315156,12.1620634870285));
#76687=CARTESIAN_POINT('Ctrl Pts',(0.744754606260194,1.49538834431159,12.185006400522));
#76688=CARTESIAN_POINT('Ctrl Pts',(0.936522631770819,1.90527961517333,12.207883870885));
#76689=CARTESIAN_POINT('Ctrl Pts',(0.91881495290156,2.35618381608074,12.2306971148174));
#76690=CARTESIAN_POINT('Ctrl Pts',(0.696757628070805,2.74758982982809,12.2534467581132));
#76691=CARTESIAN_POINT('Ctrl Pts',(0.320833811302139,2.99270696188793,12.2761349035034));
#76692=CARTESIAN_POINT('Ctrl Pts',(-0.124410755624645,3.03790832724789,
12.2987604893976));
#76693=CARTESIAN_POINT('Ctrl Pts',(-0.539746151577512,2.87395543188906,
12.3213296615096));
#76694=CARTESIAN_POINT('Ctrl Pts',(-0.783698509639943,2.59482193107452,
12.3400818248544));
#76695=CARTESIAN_POINT('Ctrl Pts',(-0.885939222791815,2.32279867038604,
12.3550664384198));
#76696=CARTESIAN_POINT('Ctrl Pts',(-0.903545681379915,2.18053231680427,
12.3625321136959));
#76697=CARTESIAN_POINT('Ctrl Pts',(-0.903850662021443,2.10752472519568,
12.3662864655665));
#76698=CARTESIAN_POINT('Ctrl Pts',(1.01808846413663,2.1,9.40201563814839));
#76699=CARTESIAN_POINT('Ctrl Pts',(1.01849147315277,2.18187084999355,9.4062191032581));
#76700=CARTESIAN_POINT('Ctrl Pts',(1.00016468627035,2.3426709426765,9.41464624341828));
#76701=CARTESIAN_POINT('Ctrl Pts',(0.887959809092518,2.64978712715063,9.43151018353515));
#76702=CARTESIAN_POINT('Ctrl Pts',(0.616026983517424,2.96710958003378,9.45264823379221));
#76703=CARTESIAN_POINT('Ctrl Pts',(0.149681573429148,3.15618792747452,9.47808179434013));
#76704=CARTESIAN_POINT('Ctrl Pts',(-0.352742227679569,3.10999193585024,
9.50359165643347));
#76705=CARTESIAN_POINT('Ctrl Pts',(-0.779178834210184,2.83755635812446,
9.52917339308576));
#76706=CARTESIAN_POINT('Ctrl Pts',(-1.03368228547638,2.39854156595712,9.55482813234504));
#76707=CARTESIAN_POINT('Ctrl Pts',(-1.05836131638902,1.89026860758708,9.58055443664554));
#76708=CARTESIAN_POINT('Ctrl Pts',(-0.846398546230643,1.42609608037824,
9.60635194366284));
#76709=CARTESIAN_POINT('Ctrl Pts',(-0.443933659380153,1.11013820065356,
9.63221975165276));
#76710=CARTESIAN_POINT('Ctrl Pts',(0.060006795418124,1.01391119317184,9.65815713286428));
#76711=CARTESIAN_POINT('Ctrl Pts',(0.553199930523459,1.16010058198549,9.68416322309809));
#76712=CARTESIAN_POINT('Ctrl Pts',(0.925230037674651,1.51732024200242,9.71023712611624));
#76713=CARTESIAN_POINT('Ctrl Pts',(1.09223473206028,2.00662699744739,9.73637791838438));
#76714=CARTESIAN_POINT('Ctrl Pts',(1.01578661403362,2.51946066235026,9.7625845501904));
#76715=CARTESIAN_POINT('Ctrl Pts',(0.711807865852075,2.94065805894325,9.78885616674331));
#76716=CARTESIAN_POINT('Ctrl Pts',(0.195466465705237,3.20300136333676,9.81811742809755));
#76717=CARTESIAN_POINT('Ctrl Pts',(-0.454284428104067,3.14688041935705,
9.85039646117044));
#76718=CARTESIAN_POINT('Ctrl Pts',(-0.990904714535579,2.67389174673884,
9.88571961297832));
#76719=CARTESIAN_POINT('Ctrl Pts',(-1.11525049429439,2.0905406551952,9.91524168134052));
#76720=CARTESIAN_POINT('Ctrl Pts',(-0.993670801030545,1.64585078282452,
9.93890924685948));
#76721=CARTESIAN_POINT('Ctrl Pts',(-0.803398272469515,1.35680145571654,
9.95668588659143));
#76722=CARTESIAN_POINT('Ctrl Pts',(-0.53159624646191,1.1419345970454,9.9744877201366));
#76723=CARTESIAN_POINT('Ctrl Pts',(-0.0971947775474125,0.981435858570208,
9.99825497858405));
#76724=CARTESIAN_POINT('Ctrl Pts',(0.419876807688296,1.04636718067241,10.0240633709415));
#76725=CARTESIAN_POINT('Ctrl Pts',(0.854104544531309,1.3805764433043,10.0519092585744));
#76726=CARTESIAN_POINT('Ctrl Pts',(1.07618290863117,1.79461751641221,10.0758179007607));
#76727=CARTESIAN_POINT('Ctrl Pts',(1.10564735137013,2.22550932349764,10.0977724598916));
#76728=CARTESIAN_POINT('Ctrl Pts',(0.989379762615938,2.59666957522658,10.1177580068108));
#76729=CARTESIAN_POINT('Ctrl Pts',(0.718140672799282,2.97766165579312,10.1417684970196));
#76730=CARTESIAN_POINT('Ctrl Pts',(0.177586859431589,3.25534176641867,10.1718391004231));
#76731=CARTESIAN_POINT('Ctrl Pts',(-0.544435702047864,3.13714319493199,
10.2080002287153));
#76732=CARTESIAN_POINT('Ctrl Pts',(-1.05596381191167,2.61253695386886,10.2442383709031));
#76733=CARTESIAN_POINT('Ctrl Pts',(-1.15623610986888,1.88502159145336,10.2805478018072));
#76734=CARTESIAN_POINT('Ctrl Pts',(-0.804336483382359,1.23911640326094,
10.3169262073463));
#76735=CARTESIAN_POINT('Ctrl Pts',(-0.136064293128745,0.927548352344434,
10.3533681275973));
#76736=CARTESIAN_POINT('Ctrl Pts',(0.506589586259768,1.05829532972237,10.3858164770831));
#76737=CARTESIAN_POINT('Ctrl Pts',(0.922867748799537,1.43166467517946,10.4142415645016));
#76738=CARTESIAN_POINT('Ctrl Pts',(1.11730226007746,1.86981865291231,10.438630689779));
#76739=CARTESIAN_POINT('Ctrl Pts',(1.11403495869486,2.34983756540438,10.4630417784934));
#76740=CARTESIAN_POINT('Ctrl Pts',(0.913723012313798,2.78652223706922,10.4874730015013));
#76741=CARTESIAN_POINT('Ctrl Pts',(0.551021545416392,3.10182228274919,10.5119244230016));
#76742=CARTESIAN_POINT('Ctrl Pts',(0.013529462665198,3.26453500307753,10.5404732227107));
#76743=CARTESIAN_POINT('Ctrl Pts',(-0.628149467334066,3.10992083738902,
10.5731348155084));
#76744=CARTESIAN_POINT('Ctrl Pts',(-1.10657260761457,2.54025825386416,10.6099062024022));
#76745=CARTESIAN_POINT('Ctrl Pts',(-1.15226055649189,1.79710936281507,10.6467151568618));
#76746=CARTESIAN_POINT('Ctrl Pts',(-0.748039471794684,1.17173686798412,
10.6835472472171));
#76747=CARTESIAN_POINT('Ctrl Pts',(-0.0504322098357749,0.908172355319504,
10.7204008353388));
#76748=CARTESIAN_POINT('Ctrl Pts',(0.587022329317992,1.08860382749987,10.7531780000451));
#76749=CARTESIAN_POINT('Ctrl Pts',(0.977623526768163,1.49569753576227,10.7818595776347));
#76750=CARTESIAN_POINT('Ctrl Pts',(1.11310778908442,1.87497891739192,10.8023509990786));
#76751=CARTESIAN_POINT('Ctrl Pts',(1.12046223639042,2.19187203555034,10.8187452228828));
#76752=CARTESIAN_POINT('Ctrl Pts',(1.05212955853369,2.55551285791366,10.8378724581563));
#76753=CARTESIAN_POINT('Ctrl Pts',(0.828422471948326,2.89870154904047,10.8583706541313));
#76754=CARTESIAN_POINT('Ctrl Pts',(0.426210055904798,3.15660019807515,10.882962075538));
#76755=CARTESIAN_POINT('Ctrl Pts',(0.00684383801692521,3.24968595364557,
10.9048257846384));
#76756=CARTESIAN_POINT('Ctrl Pts',(-0.466666320548942,3.15068796905064,
10.9294144771045));
#76757=CARTESIAN_POINT('Ctrl Pts',(-0.856906713548406,2.86577133671657,
10.9540037275576));
#76758=CARTESIAN_POINT('Ctrl Pts',(-1.13638351667166,2.37565790313556,10.9826820301581));
#76759=CARTESIAN_POINT('Ctrl Pts',(-1.12833605417664,1.71342840453131,11.0154509173227));
#76760=CARTESIAN_POINT('Ctrl Pts',(-0.677747788827833,1.11953149901379,
11.0522941233115));
#76761=CARTESIAN_POINT('Ctrl Pts',(0.0365114000399167,0.909493602222418,
11.089114442782));
#76762=CARTESIAN_POINT('Ctrl Pts',(0.735632783038763,1.16438673028385,11.1259060987032));
#76763=CARTESIAN_POINT('Ctrl Pts',(1.14626123588364,1.78418254458883,11.1626653494639));
#76764=CARTESIAN_POINT('Ctrl Pts',(1.10878693579106,2.52576163259184,11.199387935191));
#76765=CARTESIAN_POINT('Ctrl Pts',(0.638505315593813,3.09994605928972,11.2360689579805));
#76766=CARTESIAN_POINT('Ctrl Pts',(0.000388937624618915,3.26127843969028,
11.2686352489648));
#76767=CARTESIAN_POINT('Ctrl Pts',(-0.537295130790837,3.10515441545699,
11.2970961241536));
#76768=CARTESIAN_POINT('Ctrl Pts',(-0.902326569558736,2.79504264556167,
11.321466686552));
#76769=CARTESIAN_POINT('Ctrl Pts',(-1.10702206613895,2.36207264168374,11.3458150885241));
#76770=CARTESIAN_POINT('Ctrl Pts',(-1.11582534620937,1.88404100367201,11.3701349236063));
#76771=CARTESIAN_POINT('Ctrl Pts',(-0.92714626992851,1.44502786548751,11.3944306657383));
#76772=CARTESIAN_POINT('Ctrl Pts',(-0.575234030805921,1.12296279796943,
11.4186966137304));
#76773=CARTESIAN_POINT('Ctrl Pts',(-0.122301439670659,0.974089924588524,
11.4429344521201));
#76774=CARTESIAN_POINT('Ctrl Pts',(0.350698910575724,1.02504698840166,11.4671397665887));
#76775=CARTESIAN_POINT('Ctrl Pts',(0.829626204585101,1.30502543792218,11.4953420353212));
#76776=CARTESIAN_POINT('Ctrl Pts',(1.14797444119283,1.87226857357097,11.5275224305495));
#76777=CARTESIAN_POINT('Ctrl Pts',(1.05633168246765,2.59750084748831,11.5636455196149));
#76778=CARTESIAN_POINT('Ctrl Pts',(0.553638646075477,3.1250179729032,11.5996873965931));
#76779=CARTESIAN_POINT('Ctrl Pts',(-0.162948539643825,3.25108529062911,
11.6356449906589));
#76780=CARTESIAN_POINT('Ctrl Pts',(-0.811875649077865,2.92712517435771,
11.6715113968855));
#76781=CARTESIAN_POINT('Ctrl Pts',(-1.14156475071156,2.28295218061495,11.7072878404216));
#76782=CARTESIAN_POINT('Ctrl Pts',(-1.02457300660032,1.57095426196459,11.7429684336749));
#76783=CARTESIAN_POINT('Ctrl Pts',(-0.50896482368733,1.06845768586892,11.7785514654893));
#76784=CARTESIAN_POINT('Ctrl Pts',(0.201950061013787,0.971635667064493,
11.8140308939266));
#76785=CARTESIAN_POINT('Ctrl Pts',(0.830092077866532,1.31418559574247,11.8494070790025));
#76786=CARTESIAN_POINT('Ctrl Pts',(1.13102929259564,1.96096587182398,11.8846756079773));
#76787=CARTESIAN_POINT('Ctrl Pts',(0.989640144721045,2.65772453000089,11.9198339961118));
#76788=CARTESIAN_POINT('Ctrl Pts',(0.463528782418964,3.13318244291783,11.9548794729567));
#76789=CARTESIAN_POINT('Ctrl Pts',(-0.180643818085227,3.19657377969004,
11.9868989323603));
#76790=CARTESIAN_POINT('Ctrl Pts',(-0.695759946330833,2.94245729787198,
12.0159212297607));
#76791=CARTESIAN_POINT('Ctrl Pts',(-1.00225603443216,2.52836906250513,12.0419741998133));
#76792=CARTESIAN_POINT('Ctrl Pts',(-1.0841398197529,2.02076436880105,12.067959038582));
#76793=CARTESIAN_POINT('Ctrl Pts',(-0.924413211899146,1.53365759447729,
12.0938749146687));
#76794=CARTESIAN_POINT('Ctrl Pts',(-0.559890490376635,1.17509145179636,
12.1197209721359));
#76795=CARTESIAN_POINT('Ctrl Pts',(-0.072807828290282,1.02427278181782,
12.1454964045519));
#76796=CARTESIAN_POINT('Ctrl Pts',(0.427779769373155,1.11357160449807,12.1712004795833));
#76797=CARTESIAN_POINT('Ctrl Pts',(0.830406625455885,1.42180327791402,12.1968324522623));
#76798=CARTESIAN_POINT('Ctrl Pts',(1.04604179276681,1.87914271463228,12.2223917784092));
#76799=CARTESIAN_POINT('Ctrl Pts',(1.0277660461579,2.38298464567033,12.2478776032662));
#76800=CARTESIAN_POINT('Ctrl Pts',(0.781008026681809,2.8209661818624,12.2732899139927));
#76801=CARTESIAN_POINT('Ctrl Pts',(0.361964742171805,3.09601225930596,12.2986269545876));
#76802=CARTESIAN_POINT('Ctrl Pts',(-0.135051905121615,3.14792186037528,
12.3238910279141));
#76803=CARTESIAN_POINT('Ctrl Pts',(-0.599169179978984,2.96639048631031,
12.3490755266133));
#76804=CARTESIAN_POINT('Ctrl Pts',(-0.872329085896608,2.65555401105702,
12.3700076951713));
#76805=CARTESIAN_POINT('Ctrl Pts',(-0.987186930662794,2.35280215564241,
12.3867018682132));
#76806=CARTESIAN_POINT('Ctrl Pts',(-1.00734475680216,2.1938536174253,12.3950458365239));
#76807=CARTESIAN_POINT('Ctrl Pts',(-1.00792254912715,2.11275466044563,12.399218420322));
#76808=CARTESIAN_POINT('Ctrl Pts',(0.91151736992197,2.1,9.42670848231352));
#76809=CARTESIAN_POINT('Ctrl Pts',(0.911823420998916,2.17362491053193,9.43048908397653));
#76810=CARTESIAN_POINT('Ctrl Pts',(0.895347124119438,2.31730678590831,9.43801854237646));
#76811=CARTESIAN_POINT('Ctrl Pts',(0.794579867967047,2.59257652833862,9.45313636445175));
#76812=CARTESIAN_POINT('Ctrl Pts',(0.550963083297487,2.87631544921428,9.47204749845912));
#76813=CARTESIAN_POINT('Ctrl Pts',(0.133338376315858,3.04534834085169,9.49481696675561));
#76814=CARTESIAN_POINT('Ctrl Pts',(-0.316337071035398,3.00360019165658,
9.51764429868788));
#76815=CARTESIAN_POINT('Ctrl Pts',(-0.697852287982864,2.75946460258789,
9.54053895344277));
#76816=CARTESIAN_POINT('Ctrl Pts',(-0.92536205909537,2.36630063622663,9.56349815370946));
#76817=CARTESIAN_POINT('Ctrl Pts',(-0.947113368346999,1.91126111235727,
9.58652454997213));
#76818=CARTESIAN_POINT('Ctrl Pts',(-0.757015060211982,1.49578039572229,
9.60961831114713));
#76819=CARTESIAN_POINT('Ctrl Pts',(-0.396358747913306,1.21306670653134,
9.63278064943303));
#76820=CARTESIAN_POINT('Ctrl Pts',(0.0551732428288623,1.12718000131706,
9.65601225612881));
#76821=CARTESIAN_POINT('Ctrl Pts',(0.49708518307227,1.25850738740212,9.67931399514674));
#76822=CARTESIAN_POINT('Ctrl Pts',(0.830423146364994,1.57902226351323,9.70268662125709));
#76823=CARTESIAN_POINT('Ctrl Pts',(0.979930563037809,2.01805620160245,9.72613085605719));
#76824=CARTESIAN_POINT('Ctrl Pts',(0.910998864375581,2.47830509041408,9.7496474409599));
#76825=CARTESIAN_POINT('Ctrl Pts',(0.637734783618045,2.85640303606092,9.77323687378395));
#76826=CARTESIAN_POINT('Ctrl Pts',(0.173523797700195,3.09187348306677,9.79952935747188));
#76827=CARTESIAN_POINT('Ctrl Pts',(-0.410880580350844,3.0410434612312,9.82855484641837));
#76828=CARTESIAN_POINT('Ctrl Pts',(-0.893848108644005,2.61486947154893,
9.86035120685577));
#76829=CARTESIAN_POINT('Ctrl Pts',(-1.00564790149701,2.08885706686107,9.88696162003044));
#76830=CARTESIAN_POINT('Ctrl Pts',(-0.895641403689991,1.68759787522274,
9.90831870119292));
#76831=CARTESIAN_POINT('Ctrl Pts',(-0.723619481364688,1.42668451757006,
9.92436981039727));
#76832=CARTESIAN_POINT('Ctrl Pts',(-0.477850636379282,1.23267673421399,
9.94045464349453));
#76833=CARTESIAN_POINT('Ctrl Pts',(-0.0848771837976218,1.08780369054343,
9.96194746341766));
#76834=CARTESIAN_POINT('Ctrl Pts',(0.383154730739405,1.14683810870481,9.98529839642391));
#76835=CARTESIAN_POINT('Ctrl Pts',(0.776637852479867,1.45010231186482,10.0105410364593));
#76836=CARTESIAN_POINT('Ctrl Pts',(0.977937556035125,1.82603682057697,10.0322382469778));
#76837=CARTESIAN_POINT('Ctrl Pts',(1.00444635088653,2.2175629630189,10.0521814854967));
#76838=CARTESIAN_POINT('Ctrl Pts',(0.898438243730871,2.55509140919191,10.0703571117377));
#76839=CARTESIAN_POINT('Ctrl Pts',(0.651244318262303,2.90177081482339,10.0922139208646));
#76840=CARTESIAN_POINT('Ctrl Pts',(0.158339685169272,3.15464181054521,10.1196160727346));
#76841=CARTESIAN_POINT('Ctrl Pts',(-0.501122892267541,3.04634299070764,
10.1526379701481));
#76842=CARTESIAN_POINT('Ctrl Pts',(-0.969070720895698,2.56593515914924,
10.1857954825801));
#76843=CARTESIAN_POINT('Ctrl Pts',(-1.06071133600343,1.8985992051744,10.2190895515771));
#76844=CARTESIAN_POINT('Ctrl Pts',(-0.736953419031971,1.30502857084314,
10.2525184902282));
#76845=CARTESIAN_POINT('Ctrl Pts',(-0.121148835224608,1.01827893534673,
10.2860825462925));
#76846=CARTESIAN_POINT('Ctrl Pts',(0.47221947385328,1.13929533837934,10.3160345510646));
#76847=CARTESIAN_POINT('Ctrl Pts',(0.857163625188424,1.48504003896708,10.342331316347));
#76848=CARTESIAN_POINT('Ctrl Pts',(1.03707230738368,1.89123285220792,10.3649291186041));
#76849=CARTESIAN_POINT('Ctrl Pts',(1.03371636024308,2.33683112285088,10.3875856008764));
#76850=CARTESIAN_POINT('Ctrl Pts',(0.847165070768552,2.74276914283382,10.4103006996458));
#76851=CARTESIAN_POINT('Ctrl Pts',(0.509096081609499,3.03621370669456,10.4330730167258));
#76852=CARTESIAN_POINT('Ctrl Pts',(0.00747313066928684,3.18768097202426,
10.4597069040333));
#76853=CARTESIAN_POINT('Ctrl Pts',(-0.592445775936991,3.04278169853641,
10.4902356001833));
#76854=CARTESIAN_POINT('Ctrl Pts',(-1.04079931784978,2.50841253236762,10.5247114910065));
#76855=CARTESIAN_POINT('Ctrl Pts',(-1.08338436932414,1.80968101920642,10.5593052753001));
#76856=CARTESIAN_POINT('Ctrl Pts',(-0.70198015959148,1.22024016156732,10.5940225156454));
#76857=CARTESIAN_POINT('Ctrl Pts',(-0.0422454376537824,0.971372674300962,
10.6288588284583));
#76858=CARTESIAN_POINT('Ctrl Pts',(0.562108044450436,1.14276665195793,10.6599259800063));
#76859=CARTESIAN_POINT('Ctrl Pts',(0.933125339905673,1.53006298438199,10.6871887581118));
#76860=CARTESIAN_POINT('Ctrl Pts',(1.06188618556298,1.89141140995871,10.7067031606361));
#76861=CARTESIAN_POINT('Ctrl Pts',(1.06861205324963,2.19370567757229,10.7223396178189));
#76862=CARTESIAN_POINT('Ctrl Pts',(1.00304025429932,2.54085849191131,10.7406013583902));
#76863=CARTESIAN_POINT('Ctrl Pts',(0.78883783544409,2.86897570776504,10.760201975507));
#76864=CARTESIAN_POINT('Ctrl Pts',(0.403053119117575,3.11584641273972,10.7837746681186));
#76865=CARTESIAN_POINT('Ctrl Pts',(0.000362036933634016,3.20485996514675,
10.8047589130325));
#76866=CARTESIAN_POINT('Ctrl Pts',(-0.455152490817227,3.10924210303583,
10.8284161801311));
#76867=CARTESIAN_POINT('Ctrl Pts',(-0.831125997851916,2.83422752561369,
10.8521153778398));
#76868=CARTESIAN_POINT('Ctrl Pts',(-1.10072731360356,2.36050560413651,10.8798183647944));
#76869=CARTESIAN_POINT('Ctrl Pts',(-1.09252964318303,1.71909233641417,10.9115478665288));
#76870=CARTESIAN_POINT('Ctrl Pts',(-0.654361811393719,1.14228170583733,
10.9473395695622));
#76871=CARTESIAN_POINT('Ctrl Pts',(0.0420042139168913,0.937977236263047,
10.983221779786));
#76872=CARTESIAN_POINT('Ctrl Pts',(0.725507027710317,1.18765705960442,11.0191917529181));
#76873=CARTESIAN_POINT('Ctrl Pts',(1.12796260215576,1.79594785111174,11.055245666088));
#76874=CARTESIAN_POINT('Ctrl Pts',(1.09061376681782,2.52577506847939,11.0913797672831));
#76875=CARTESIAN_POINT('Ctrl Pts',(0.625902914242613,3.09240832046028,11.1275906675829));
#76876=CARTESIAN_POINT('Ctrl Pts',(-0.00630633598939572,3.25178721005664,
11.1598420116462));
#76877=CARTESIAN_POINT('Ctrl Pts',(-0.540240864569795,3.09619033576691,
11.1881081914955));
#76878=CARTESIAN_POINT('Ctrl Pts',(-0.903308708901617,2.78712934837545,
11.2123665462451));
#76879=CARTESIAN_POINT('Ctrl Pts',(-1.10707609254612,2.35500603102821,11.2366515647841));
#76880=CARTESIAN_POINT('Ctrl Pts',(-1.11540058169363,1.87706321585021,11.2609655395252));
#76881=CARTESIAN_POINT('Ctrl Pts',(-0.925908271596444,1.43740578510329,
11.285303445506));
#76882=CARTESIAN_POINT('Ctrl Pts',(-0.572210730312777,1.11438275513905,
11.309667110669));
#76883=CARTESIAN_POINT('Ctrl Pts',(-0.116275510175771,0.965056470550933,
11.3340534145616));
#76884=CARTESIAN_POINT('Ctrl Pts',(0.360700243291035,1.01696185361064,11.3584631352109));
#76885=CARTESIAN_POINT('Ctrl Pts',(0.844446227881871,1.30044236766626,11.3869657989611));
#76886=CARTESIAN_POINT('Ctrl Pts',(1.16657608619672,1.87553441489441,11.4195706490173));
#76887=CARTESIAN_POINT('Ctrl Pts',(1.07280974558895,2.61279947948096,11.4562923059314));
#76888=CARTESIAN_POINT('Ctrl Pts',(0.55961199987561,3.15041796179706,11.4930495823791));
#76889=CARTESIAN_POINT('Ctrl Pts',(-0.173736551317003,3.27879187689283,
11.5298376714367));
#76890=CARTESIAN_POINT('Ctrl Pts',(-0.839605484416093,2.94563868032413,
11.5666541180967));
#76891=CARTESIAN_POINT('Ctrl Pts',(-1.17851839519367,2.28198286935752,11.603492067794));
#76892=CARTESIAN_POINT('Ctrl Pts',(-1.0569823061534,1.54658256971973,11.640348201911));
#76893=CARTESIAN_POINT('Ctrl Pts',(-0.522199558365981,1.02637377533744,
11.6772175075259));
#76894=CARTESIAN_POINT('Ctrl Pts',(0.216893871560646,0.926443560152882,
11.7140965345869));
#76895=CARTESIAN_POINT('Ctrl Pts',(0.871476025423946,1.28425104909088,11.7509795818237));
#76896=CARTESIAN_POINT('Ctrl Pts',(1.18551994913662,1.96099154468725,11.787862507617));
#76897=CARTESIAN_POINT('Ctrl Pts',(1.03644815019712,2.69171293013048,11.824740942292));
#76898=CARTESIAN_POINT('Ctrl Pts',(0.482409520039158,3.19134922941584,11.8616103433384));
#76899=CARTESIAN_POINT('Ctrl Pts',(-0.197372192715649,3.25749187034555,
11.8953948352799));
#76900=CARTESIAN_POINT('Ctrl Pts',(-0.741930590032224,2.98797239484732,
11.926094816338));
#76901=CARTESIAN_POINT('Ctrl Pts',(-1.06625417361505,2.54857764239091,11.9537127158612));
#76902=CARTESIAN_POINT('Ctrl Pts',(-1.15252001058213,2.00922868658725,11.9813166994033));
#76903=CARTESIAN_POINT('Ctrl Pts',(-0.981783734819453,1.49092372364447,
12.008904888169));
#76904=CARTESIAN_POINT('Ctrl Pts',(-0.592420461199662,1.10897317214394,
12.036475439748));
#76905=CARTESIAN_POINT('Ctrl Pts',(-0.071571264224261,0.948492450725194,
12.0640264518274));
#76906=CARTESIAN_POINT('Ctrl Pts',(0.464419135236049,1.04488560113194,12.091556134534));
#76907=CARTESIAN_POINT('Ctrl Pts',(0.89600235444067,1.37626327825661,12.1190625678794));
#76908=CARTESIAN_POINT('Ctrl Pts',(1.12713249773057,1.86831043871101,12.1465442073483));
#76909=CARTESIAN_POINT('Ctrl Pts',(1.10664927335543,2.41102174199376,12.1739987168217));
#76910=CARTESIAN_POINT('Ctrl Pts',(0.839640517933186,2.88329040026059,12.2014255755425));
#76911=CARTESIAN_POINT('Ctrl Pts',(0.386132852406335,3.17999397807018,12.2288202203781));
#76912=CARTESIAN_POINT('Ctrl Pts',(-0.152290410197637,3.23536449519144,
12.2561871890178));
#76913=CARTESIAN_POINT('Ctrl Pts',(-0.655550821832348,3.03769445607198,
12.2835107392738));
#76914=CARTESIAN_POINT('Ctrl Pts',(-0.951961764434413,2.69925795049044,
12.3062694694656));
#76915=CARTESIAN_POINT('Ctrl Pts',(-1.07634979864707,2.36980477421791,12.3244258281199));
#76916=CARTESIAN_POINT('Ctrl Pts',(-1.09803441854211,2.1963840236327,12.3335275999414));
#76917=CARTESIAN_POINT('Ctrl Pts',(-1.09851387392196,2.10832492681077,12.3380569618133));
#76918=CARTESIAN_POINT('Ctrl Pts',(0.88,2.1,9.49208807696239));
#76919=CARTESIAN_POINT('Ctrl Pts',(0.88004530066288,2.17110443853451,9.49574149503588));
#76920=CARTESIAN_POINT('Ctrl Pts',(0.863615235646394,2.30953923705568,9.50300212441786));
#76921=CARTESIAN_POINT('Ctrl Pts',(0.765462544235921,2.57462340525805,9.51758083803204));
#76922=CARTESIAN_POINT('Ctrl Pts',(0.529819591157008,2.84681044164821,9.5357938837476));
#76923=CARTESIAN_POINT('Ctrl Pts',(0.12778461713841,3.00776193746932,9.55768645918373));
#76924=CARTESIAN_POINT('Ctrl Pts',(-0.303559189553242,2.96604809729294,
9.57959800515177));
#76925=CARTESIAN_POINT('Ctrl Pts',(-0.668168144789344,2.7308027674258,9.60153880818797));
#76926=CARTESIAN_POINT('Ctrl Pts',(-0.884366875518534,2.35394413226399,
9.62350665193357));
#76927=CARTESIAN_POINT('Ctrl Pts',(-0.90352025454572,1.91932181682493,9.6455048808308));
#76928=CARTESIAN_POINT('Ctrl Pts',(-0.72078437125489,1.52382494797329,9.66753430657136));
#76929=CARTESIAN_POINT('Ctrl Pts',(-0.376394911298066,1.25592019629859,
9.68959681841591));
#76930=CARTESIAN_POINT('Ctrl Pts',(0.0532124427449469,1.17584944736387,
9.71169377532346));
#76931=CARTESIAN_POINT('Ctrl Pts',(0.472332248812248,1.30208619516318,9.73382675522453));
#76932=CARTESIAN_POINT('Ctrl Pts',(0.787286422179607,1.60715424951494,9.75599718708746));
#76933=CARTESIAN_POINT('Ctrl Pts',(0.927347587472474,2.02341832269235,9.77820662437522));
#76934=CARTESIAN_POINT('Ctrl Pts',(0.860575112492045,2.4584680844061,9.80045633596402));
#76935=CARTESIAN_POINT('Ctrl Pts',(0.601155266029929,2.81469328323033,9.82274803545432));
#76936=CARTESIAN_POINT('Ctrl Pts',(0.162372489010935,3.0352765216471,9.84756385390868));
#76937=CARTESIAN_POINT('Ctrl Pts',(-0.388150801165923,2.98535810090146,
9.87492859407763));
#76938=CARTESIAN_POINT('Ctrl Pts',(-0.841141613414809,2.58266182781169,
9.90486455365364));
#76939=CARTESIAN_POINT('Ctrl Pts',(-0.944423152013141,2.08801695854391,
9.92987876914174));
#76940=CARTESIAN_POINT('Ctrl Pts',(-0.839850650288727,1.71170647032559,
9.94993165014419));
#76941=CARTESIAN_POINT('Ctrl Pts',(-0.677623291964419,1.46747623780434,
9.96499472728963));
#76942=CARTESIAN_POINT('Ctrl Pts',(-0.44655290394383,1.28636379874863,9.98008084963806));
#76943=CARTESIAN_POINT('Ctrl Pts',(-0.0778471165786419,1.15186841586681,
10.0002245579097));
#76944=CARTESIAN_POINT('Ctrl Pts',(0.360306690446967,1.20869984432036,10.0221099156808));
#76945=CARTESIAN_POINT('Ctrl Pts',(0.727434680359908,1.49366178825316,10.0457287929528));
#76946=CARTESIAN_POINT('Ctrl Pts',(0.914446196367802,1.84575615010426,10.0660175354139));
#76947=CARTESIAN_POINT('Ctrl Pts',(0.937977426449006,2.21168850001371,10.0846590915643));
#76948=CARTESIAN_POINT('Ctrl Pts',(0.837928158967066,2.52657011588598,10.1016371890881));
#76949=CARTESIAN_POINT('Ctrl Pts',(0.606093172372672,2.84942473726904,10.122044518861));
#76950=CARTESIAN_POINT('Ctrl Pts',(0.145376230198328,3.08381718275388,10.147626054432));
#76951=CARTESIAN_POINT('Ctrl Pts',(-0.46914671489129,2.98076716295159,10.1784259790307));
#76952=CARTESIAN_POINT('Ctrl Pts',(-0.903690880659961,2.53167055598801,
10.2093356131282));
#76953=CARTESIAN_POINT('Ctrl Pts',(-0.986972114311235,1.90988467649814,
10.2403547285203));
#76954=CARTESIAN_POINT('Ctrl Pts',(-0.683752522804138,1.35832101547673,
10.2714868311644));
#76955=CARTESIAN_POINT('Ctrl Pts',(-0.109813487751821,1.09335411156601,
10.3027322600927));
#76956=CARTESIAN_POINT('Ctrl Pts',(0.441878190810725,1.20774702806893,10.3306109818244));
#76957=CARTESIAN_POINT('Ctrl Pts',(0.798907968654179,1.53050023949423,10.3550769566962));
#76958=CARTESIAN_POINT('Ctrl Pts',(0.965032703288519,1.90884357252065,10.3761014912007));
#76959=CARTESIAN_POINT('Ctrl Pts',(0.960597360585514,2.323268162612,10.3971783739586));
#76960=CARTESIAN_POINT('Ctrl Pts',(0.785897643856786,2.70024077531878,10.4183074156142));
#76961=CARTESIAN_POINT('Ctrl Pts',(0.470625209333448,2.97216502173762,10.4394903861049));
#76962=CARTESIAN_POINT('Ctrl Pts',(0.00362841706809864,3.11156549341437,
10.4642669695311));
#76963=CARTESIAN_POINT('Ctrl Pts',(-0.554041350695444,2.97505278451906,
10.492678523291));
#76964=CARTESIAN_POINT('Ctrl Pts',(-0.969608931768246,2.47660542892771,
10.5247571910533));
#76965=CARTESIAN_POINT('Ctrl Pts',(-1.00726653710962,1.82619792265918,10.5569658388182));
#76966=CARTESIAN_POINT('Ctrl Pts',(-0.65050065906872,1.27853344965516,10.5892959338387));
#76967=CARTESIAN_POINT('Ctrl Pts',(-0.035343368509533,1.04859916693606,
10.6217508876492));
#76968=CARTESIAN_POINT('Ctrl Pts',(0.527368249504387,1.21002444550603,10.6507128983937));
#76969=CARTESIAN_POINT('Ctrl Pts',(0.872149475938407,1.57212693960115,10.6761311036372));
#76970=CARTESIAN_POINT('Ctrl Pts',(0.991208146851818,1.90950718557218,10.6943339612799));
#76971=CARTESIAN_POINT('Ctrl Pts',(0.996618420282601,2.19155347984175,10.7089238607875));
#76972=CARTESIAN_POINT('Ctrl Pts',(0.934433485677006,2.51531393887681,10.7259668475802));
#76973=CARTESIAN_POINT('Ctrl Pts',(0.733532233043949,2.8210729242721,10.7442719027377));
#76974=CARTESIAN_POINT('Ctrl Pts',(0.372500390277194,3.05055151027295,10.7662896596735));
#76975=CARTESIAN_POINT('Ctrl Pts',(-0.00407736089083116,3.13262070332373,
10.7859052812708));
#76976=CARTESIAN_POINT('Ctrl Pts',(-0.429697688628497,3.04193960479491,
10.808025020752));
#76977=CARTESIAN_POINT('Ctrl Pts',(-0.780690595728469,2.78360253048668,
10.8302023050984));
#76978=CARTESIAN_POINT('Ctrl Pts',(-1.0317479290845,2.33939629334436,10.8561382785999));
#76979=CARTESIAN_POINT('Ctrl Pts',(-1.02235302842942,1.73847951063121,10.8858727969815));
#76980=CARTESIAN_POINT('Ctrl Pts',(-0.609877440485562,1.19869136833044,
10.9194453166195));
#76981=CARTESIAN_POINT('Ctrl Pts',(0.0444562651571831,1.00873193799866,
10.9531396787437));
#76982=CARTESIAN_POINT('Ctrl Pts',(0.686241226456731,1.24523149613666,10.9869542078945));
#76983=CARTESIAN_POINT('Ctrl Pts',(1.06336671190863,1.81874075355131,11.0208880789452));
#76984=CARTESIAN_POINT('Ctrl Pts',(1.02624403939236,2.50632313928255,11.0549398755566));
#76985=CARTESIAN_POINT('Ctrl Pts',(0.586303974101457,3.03971411671832,11.0891082207085));
#76986=CARTESIAN_POINT('Ctrl Pts',(-0.0114201944887836,3.18863269329433,
11.1195823360316));
#76987=CARTESIAN_POINT('Ctrl Pts',(-0.516038343262635,3.0399955245707,11.1463206001162));
#76988=CARTESIAN_POINT('Ctrl Pts',(-0.858934951304874,2.74638434222921,
11.1692889561686));
#76989=CARTESIAN_POINT('Ctrl Pts',(-1.05087415829708,2.33628887027357,11.1923064654593));
#76990=CARTESIAN_POINT('Ctrl Pts',(-1.05745931905409,1.88285594553982,11.2153729875302));
#76991=CARTESIAN_POINT('Ctrl Pts',(-0.87630769190474,1.46584630314957,11.2384871521497));
#76992=CARTESIAN_POINT('Ctrl Pts',(-0.539183017509096,1.15973291652138,
11.2616491583461));
#76993=CARTESIAN_POINT('Ctrl Pts',(-0.104881518069885,1.018866539415,11.2848576413368));
#76994=CARTESIAN_POINT('Ctrl Pts',(0.349386797262332,1.06962249267029,11.3081130241157));
#76995=CARTESIAN_POINT('Ctrl Pts',(0.809972444245432,1.34130820500274,11.3352974299965));
#76996=CARTESIAN_POINT('Ctrl Pts',(1.11614064498991,1.89139132293948,11.3664379798849));
#76997=CARTESIAN_POINT('Ctrl Pts',(1.02453105287773,2.59650367918193,11.4015700842448));
#76998=CARTESIAN_POINT('Ctrl Pts',(0.531295143907132,3.11042556597401,11.4367980923007));
#76999=CARTESIAN_POINT('Ctrl Pts',(-0.173129048624275,3.2317907557564,11.4721176408173));
#77000=CARTESIAN_POINT('Ctrl Pts',(-0.812751586742188,2.90961035470477,
11.5075304282483));
#77001=CARTESIAN_POINT('Ctrl Pts',(-1.13763474000058,2.26920222604431,11.5430275630626));
#77002=CARTESIAN_POINT('Ctrl Pts',(-1.0183897866875,1.55950706457121,11.5786099463847));
#77003=CARTESIAN_POINT('Ctrl Pts',(-0.499742430458015,1.05767695948834,
11.6142714083728));
#77004=CARTESIAN_POINT('Ctrl Pts',(0.216875431514358,0.962745864867631,
11.6500148062663));
#77005=CARTESIAN_POINT('Ctrl Pts',(0.851628626733939,1.31191607717112,11.6858294674315));
#77006=CARTESIAN_POINT('Ctrl Pts',(1.15545700022636,1.97124830788862,11.721715748643));
#77007=CARTESIAN_POINT('Ctrl Pts',(1.00820496754727,2.68333851027724,11.7576694901916));
#77008=CARTESIAN_POINT('Ctrl Pts',(0.465592530984764,3.17005424157605,11.793687902103));
#77009=CARTESIAN_POINT('Ctrl Pts',(-0.200114414825182,3.23303114166232,
11.8267591746644));
#77010=CARTESIAN_POINT('Ctrl Pts',(-0.73349915290536,2.96717013530568,11.8568679625751));
#77011=CARTESIAN_POINT('Ctrl Pts',(-1.05088301096295,2.53462253501223,11.8839956498509));
#77012=CARTESIAN_POINT('Ctrl Pts',(-1.1342639661375,2.00370734901977,11.9111524047389));
#77013=CARTESIAN_POINT('Ctrl Pts',(-0.964560539044214,1.49340428201235,
11.9383363187367));
#77014=CARTESIAN_POINT('Ctrl Pts',(-0.579170342282215,1.11748888725573,
11.9655459647886));
#77015=CARTESIAN_POINT('Ctrl Pts',(-0.0637901249951442,0.960293629116356,
11.9927796193207));
#77016=CARTESIAN_POINT('Ctrl Pts',(0.466690930572303,1.05725236797281,12.0200357099596));
#77017=CARTESIAN_POINT('Ctrl Pts',(0.893812980941284,1.3871367670854,12.0473125059984));
#77018=CARTESIAN_POINT('Ctrl Pts',(1.12203809139043,1.87660228457252,12.074608533169));
#77019=CARTESIAN_POINT('Ctrl Pts',(1.10012614833113,2.41656001477662,12.1019217271321));
#77020=CARTESIAN_POINT('Ctrl Pts',(0.83268402875598,2.88648791750582,12.1292512722902));
#77021=CARTESIAN_POINT('Ctrl Pts',(0.379131566217826,3.18138175025283,12.1565934803869));
#77022=CARTESIAN_POINT('Ctrl Pts',(-0.159356724291243,3.23521048606865,
12.1839510331369));
#77023=CARTESIAN_POINT('Ctrl Pts',(-0.662789041493893,3.03578242415445,
12.211312326472));
#77024=CARTESIAN_POINT('Ctrl Pts',(-0.959078027836141,2.69544897818908,
12.2341338236766));
#77025=CARTESIAN_POINT('Ctrl Pts',(-1.08301523558641,2.36413115081123,12.2523724677113));
#77026=CARTESIAN_POINT('Ctrl Pts',(-1.10424709743569,2.18973503538251,12.2615198955416));
#77027=CARTESIAN_POINT('Ctrl Pts',(-1.10446356961415,2.10123734103367,12.2660694403094));
#77028=CARTESIAN_POINT('Ctrl Pts',(0.88,2.1,9.525));
#77029=CARTESIAN_POINT('Ctrl Pts',(0.879914606625585,2.17110785049955,9.52865476385635));
#77030=CARTESIAN_POINT('Ctrl Pts',(0.863232117186907,2.3095104036224,9.53591397312323));
#77031=CARTESIAN_POINT('Ctrl Pts',(0.7646146646842,2.57432753790838,9.55048599717583));
#77032=CARTESIAN_POINT('Ctrl Pts',(0.52875066403414,2.8457083400553,9.56867094599734));
#77033=CARTESIAN_POINT('Ctrl Pts',(0.127238756664634,3.00552936974926,9.59051359518968));
#77034=CARTESIAN_POINT('Ctrl Pts',(-0.302716205619033,2.96306288294985,
9.61235380295566));
#77035=CARTESIAN_POINT('Ctrl Pts',(-0.665427657999688,2.72799341501097,
9.63420407641812));
#77036=CARTESIAN_POINT('Ctrl Pts',(-0.879826065415376,2.3524940033895,9.65606121698024));
#77037=CARTESIAN_POINT('Ctrl Pts',(-0.89799221853441,1.92029343459682,9.67792905414005));
#77038=CARTESIAN_POINT('Ctrl Pts',(-0.715657796510551,1.52775201761214,
9.69980826165769));
#77039=CARTESIAN_POINT('Ctrl Pts',(-0.37329244035757,1.26252484692041,9.72170089413125));
#77040=CARTESIAN_POINT('Ctrl Pts',(0.0529042162174613,1.18397194405211,
9.7436083723133));
#77041=CARTESIAN_POINT('Ctrl Pts',(0.467926525737336,1.30987826775351,9.76553239226868));
#77042=CARTESIAN_POINT('Ctrl Pts',(0.77911594458734,1.61250328722602,9.78747453406851));
#77043=CARTESIAN_POINT('Ctrl Pts',(0.916833254715888,2.02450810034898,9.8094364412056));
#77044=CARTESIAN_POINT('Ctrl Pts',(0.84999015619955,2.45432327019144,9.83141968646686));
#77045=CARTESIAN_POINT('Ctrl Pts',(0.593134887517594,2.80556810401153,9.85342584950507));
#77046=CARTESIAN_POINT('Ctrl Pts',(0.159785468035136,3.02235194398505,9.87790429996245));
#77047=CARTESIAN_POINT('Ctrl Pts',(-0.382738476891779,2.97204316801605,
9.90486768286448));
#77048=CARTESIAN_POINT('Ctrl Pts',(-0.827943575417754,2.57464859578558,
9.93433214776037));
#77049=CARTESIAN_POINT('Ctrl Pts',(-0.928540642244484,2.0879125901631,9.95893043030863));
#77050=CARTESIAN_POINT('Ctrl Pts',(-0.82506221727755,1.71823863855703,9.97863755083128));
#77051=CARTESIAN_POINT('Ctrl Pts',(-0.665238898770628,1.47861418311032,
9.99343255715118));
#77052=CARTESIAN_POINT('Ctrl Pts',(-0.438025190317537,1.3012081221325,10.0082426633322));
#77053=CARTESIAN_POINT('Ctrl Pts',(-0.0759140953759721,1.16989403941721,
10.0280101634631));
#77054=CARTESIAN_POINT('Ctrl Pts',(0.353590617267489,1.22647296601624,10.0494595111079));
#77055=CARTESIAN_POINT('Ctrl Pts',(0.71282299611785,1.50640456177768,10.0726022736917));
#77056=CARTESIAN_POINT('Ctrl Pts',(0.895311256816217,1.85157831854142,10.0924697020734));
#77057=CARTESIAN_POINT('Ctrl Pts',(0.917661293713379,2.20976194577009,10.1107106042816));
#77058=CARTESIAN_POINT('Ctrl Pts',(0.819212469046223,2.51761130734418,10.127317066638));
#77059=CARTESIAN_POINT('Ctrl Pts',(0.591924394917487,2.83289082559773,10.1472698428113));
#77060=CARTESIAN_POINT('Ctrl Pts',(0.141288805504938,3.06103897732418,10.172258699084));
#77061=CARTESIAN_POINT('Ctrl Pts',(-0.458527011040082,2.95925151709148,
10.2023249565719));
#77062=CARTESIAN_POINT('Ctrl Pts',(-0.88162766536303,2.52027411449529,10.2324736532743));
#77063=CARTESIAN_POINT('Ctrl Pts',(-0.961653185964405,1.91393657438503,
10.2627077273853));
#77064=CARTESIAN_POINT('Ctrl Pts',(-0.665231767857691,1.37715957803001,
10.2930297792945));
#77065=CARTESIAN_POINT('Ctrl Pts',(-0.105988685338195,1.12026073865136,
10.3234425669733));
#77066=CARTESIAN_POINT('Ctrl Pts',(0.430538820721984,1.23255710504194,10.3505590141325));
#77067=CARTESIAN_POINT('Ctrl Pts',(0.777157271318668,1.54704609431923,10.3743479205533));
#77068=CARTESIAN_POINT('Ctrl Pts',(0.937973646848606,1.91510656924282,10.3947816504623));
#77069=CARTESIAN_POINT('Ctrl Pts',(0.932931736507626,2.31778957988939,10.4152592321293));
#77070=CARTESIAN_POINT('Ctrl Pts',(0.762578582228501,2.68366310973811,10.4357813746755));
#77071=CARTESIAN_POINT('Ctrl Pts',(0.455963235969408,2.94715653506223,10.4563486739678));
#77072=CARTESIAN_POINT('Ctrl Pts',(0.00240142086611935,3.08166579400621,
10.480397254692));
#77073=CARTESIAN_POINT('Ctrl Pts',(-0.538455390507358,2.94820992747045,
10.5079586157699));
#77074=CARTESIAN_POINT('Ctrl Pts',(-0.940666416691817,2.46401744657124,
10.5390713811047));
#77075=CARTESIAN_POINT('Ctrl Pts',(-0.976029443563649,1.83335883304997,
10.5702921359498));
#77076=CARTESIAN_POINT('Ctrl Pts',(-0.629306856593687,1.30317046301086,
10.6016225477596));
#77077=CARTESIAN_POINT('Ctrl Pts',(-0.0328763589810331,1.08144514613719,
10.6330641573791));
#77078=CARTESIAN_POINT('Ctrl Pts',(0.511901871764286,1.23876013099839,10.6611123163153));
#77079=CARTESIAN_POINT('Ctrl Pts',(0.845208777494887,1.59002857501027,10.6857282761483));
#77080=CARTESIAN_POINT('Ctrl Pts',(0.959937391714928,1.91692164410815,10.7033535735637));
#77081=CARTESIAN_POINT('Ctrl Pts',(0.964709509971458,2.19002072343591,10.7174794574177));
#77082=CARTESIAN_POINT('Ctrl Pts',(0.903969607200192,2.50338072207659,10.7339796596208));
#77083=CARTESIAN_POINT('Ctrl Pts',(0.708976511873778,2.79903473649909,10.7516978643424));
#77084=CARTESIAN_POINT('Ctrl Pts',(0.359111666410103,3.02058677865832,10.7730116718645));
#77085=CARTESIAN_POINT('Ctrl Pts',(-0.0055195068732309,3.09939687665217,
10.7919958841582));
#77086=CARTESIAN_POINT('Ctrl Pts',(-0.417331250225881,3.01093271757532,
10.8134054790171));
#77087=CARTESIAN_POINT('Ctrl Pts',(-0.756608961158023,2.76032613000462,
10.8348676292604));
#77088=CARTESIAN_POINT('Ctrl Pts',(-0.998865593098056,2.33000290793379,
10.8599683150449));
#77089=CARTESIAN_POINT('Ctrl Pts',(-0.988791187924089,1.74845036869023,
10.8887429491342));
#77090=CARTESIAN_POINT('Ctrl Pts',(-0.588714669350558,1.22669384301482,
10.9212338011637));
#77091=CARTESIAN_POINT('Ctrl Pts',(0.044909234496707,1.04388405761621,10.9538443040117));
#77092=CARTESIAN_POINT('Ctrl Pts',(0.665762350574508,1.27382859359802,10.9865746011287));
#77093=CARTESIAN_POINT('Ctrl Pts',(1.02994927065475,1.82963242200099,11.0194247010519));
#77094=CARTESIAN_POINT('Ctrl Pts',(0.99292771913683,2.49532007970257,11.0523944801788));
#77095=CARTESIAN_POINT('Ctrl Pts',(0.566047404042377,3.01118540039736,11.0854836852924));
#77096=CARTESIAN_POINT('Ctrl Pts',(-0.0131656805453273,3.1545072720966,
11.1150021335127));
#77097=CARTESIAN_POINT('Ctrl Pts',(-0.501834747536299,3.00971245930524,
11.1409075995603));
#77098=CARTESIAN_POINT('Ctrl Pts',(-0.833654637909307,2.72466132918788,
11.1631647757637));
#77099=CARTESIAN_POINT('Ctrl Pts',(-1.01904932840502,2.32688792491809,11.1854742337572));
#77100=CARTESIAN_POINT('Ctrl Pts',(-1.0247320303861,1.8873087550975,11.2078357472338));
#77101=CARTESIAN_POINT('Ctrl Pts',(-0.848433071641297,1.48323440703255,
11.2302490424206));
#77102=CARTESIAN_POINT('Ctrl Pts',(-0.5209916303453,1.18686010809674,11.2527138516101));
#77103=CARTESIAN_POINT('Ctrl Pts',(-0.0994474829318688,1.05086828612434,
11.2752298585268));
#77104=CARTESIAN_POINT('Ctrl Pts',(0.341286571712092,1.10081439784123,11.297796723956));
#77105=CARTESIAN_POINT('Ctrl Pts',(0.787934060544661,1.36522529701193,11.3241836591263));
#77106=CARTESIAN_POINT('Ctrl Pts',(1.08440822726537,1.89981767692546,11.3544236935599));
#77107=CARTESIAN_POINT('Ctrl Pts',(0.99437189083192,2.58466520846377,11.3885550724356));
#77108=CARTESIAN_POINT('Ctrl Pts',(0.51422832678732,3.08343949927552,11.4227963300144));
#77109=CARTESIAN_POINT('Ctrl Pts',(-0.170956362315584,3.20042729316684,
11.4571457685877));
#77110=CARTESIAN_POINT('Ctrl Pts',(-0.792809143568463,2.88603885152724,
11.49160167588));
#77111=CARTESIAN_POINT('Ctrl Pts',(-1.10815562220614,2.26212033857722,11.5261621918766));
#77112=CARTESIAN_POINT('Ctrl Pts',(-0.990980784814367,1.57098681332194,
11.5608252913622));
#77113=CARTESIAN_POINT('Ctrl Pts',(-0.484736723033935,1.08260154598769,
11.5955889188738));
#77114=CARTESIAN_POINT('Ctrl Pts',(0.214307763377102,0.991032096532327,
11.6304507824074));
#77115=CARTESIAN_POINT('Ctrl Pts',(0.833298379906107,1.33271197734595,11.6654086518246));
#77116=CARTESIAN_POINT('Ctrl Pts',(1.12908711130714,1.97705558535849,11.7004600148669));
#77117=CARTESIAN_POINT('Ctrl Pts',(0.984170425255086,2.67277304384029,11.7356024461146));
#77118=CARTESIAN_POINT('Ctrl Pts',(0.452808643636702,3.14802102155422,11.7708333087139));
#77119=CARTESIAN_POINT('Ctrl Pts',(-0.198836507924274,3.20872213800758,
11.8032068201948));
#77120=CARTESIAN_POINT('Ctrl Pts',(-0.720833985617695,2.9475724124579,11.8326976979388));
#77121=CARTESIAN_POINT('Ctrl Pts',(-1.03122512713103,2.52323917223077,11.8592848682016));
#77122=CARTESIAN_POINT('Ctrl Pts',(-1.11221371795246,2.00254397936835,11.8859162010712));
#77123=CARTESIAN_POINT('Ctrl Pts',(-0.944978677865563,1.50212478400673,
11.9125904181942));
#77124=CARTESIAN_POINT('Ctrl Pts',(-0.566096651435205,1.13364169683645,
11.9393062323883));
#77125=CARTESIAN_POINT('Ctrl Pts',(-0.0596069971212731,0.97996909355213,
11.966062281935));
#77126=CARTESIAN_POINT('Ctrl Pts',(0.461675051948685,1.07603593590851,11.9928572469173));
#77127=CARTESIAN_POINT('Ctrl Pts',(0.88129231323125,1.40110770643291,12.0196896905075));
#77128=CARTESIAN_POINT('Ctrl Pts',(1.10519737818586,1.88315811002375,12.0465583931276));
#77129=CARTESIAN_POINT('Ctrl Pts',(1.08283365883886,2.41488670097258,12.0734615789711));
#77130=CARTESIAN_POINT('Ctrl Pts',(0.818591168747924,2.87760074176854,12.100398642491));
#77131=CARTESIAN_POINT('Ctrl Pts',(0.370893737846914,3.16774776724325,12.1273662612715));
#77132=CARTESIAN_POINT('Ctrl Pts',(-0.160578831483255,3.22009488317826,
12.154367120808));
#77133=CARTESIAN_POINT('Ctrl Pts',(-0.657438304412148,3.02243699025829,
12.181390412703));
#77134=CARTESIAN_POINT('Ctrl Pts',(-0.949764066307816,2.68573447988004,
12.2039450357004));
#77135=CARTESIAN_POINT('Ctrl Pts',(-1.07182425162092,2.35796849387404,12.2219800536891));
#77136=CARTESIAN_POINT('Ctrl Pts',(-1.09256785760649,2.18550272007321,12.2310256553714));
#77137=CARTESIAN_POINT('Ctrl Pts',(-1.09265261173395,2.09796323888708,12.2355247810852));
#77138=CARTESIAN_POINT('',(0.88,2.1,9.525));
#77139=CARTESIAN_POINT('Ctrl Pts',(0.88,2.1,9.525));
#77140=CARTESIAN_POINT('Ctrl Pts',(0.88,2.1,9.52654752419537));
#77141=CARTESIAN_POINT('Ctrl Pts',(0.880034855304809,2.10000000001394,9.52809491473538));
#77142=CARTESIAN_POINT('Ctrl Pts',(0.880757639620712,2.10000000001394,9.54426404545797));
#77143=CARTESIAN_POINT('Ctrl Pts',(0.884474056104899,2.10000000001393,9.55873384801261));
#77144=CARTESIAN_POINT('Ctrl Pts',(0.896554877287777,2.10000000001393,9.58437291981711));
#77145=CARTESIAN_POINT('Ctrl Pts',(0.904632693604525,2.10000000001391,9.5957497323212));
#77146=CARTESIAN_POINT('Ctrl Pts',(0.926145942464148,2.10000000001391,9.61621866481436));
#77147=CARTESIAN_POINT('Ctrl Pts',(0.938680653436097,2.1000000000139,9.62308237886113));
#77148=CARTESIAN_POINT('Ctrl Pts',(0.963545489976373,2.1000000000139,9.63257445432811));
#77149=CARTESIAN_POINT('Ctrl Pts',(0.97799462547993,2.10000000001388,9.63514919539636));
#77150=CARTESIAN_POINT('Ctrl Pts',(1.00659276824775,2.10000000001388,9.6347066681337));
#77151=CARTESIAN_POINT('Ctrl Pts',(1.02034071065155,2.10000000001387,9.63174790532893));
#77152=CARTESIAN_POINT('Ctrl Pts',(1.04687463693244,2.10000000001387,9.62016351498204));
#77153=CARTESIAN_POINT('Ctrl Pts',(1.05918781850548,2.10000000001387,9.611590130133));
#77154=CARTESIAN_POINT('Ctrl Pts',(1.07740651951704,2.10000000001387,9.5928426732394));
#77155=CARTESIAN_POINT('Ctrl Pts',(1.08570485806481,2.10000000001386,9.58187096954533));
#77156=CARTESIAN_POINT('Ctrl Pts',(1.09719990931814,2.10000000001386,9.55415037431876));
#77157=CARTESIAN_POINT('Ctrl Pts',(1.09993578707158,2.10000000001386,9.53955469920238));
#77158=CARTESIAN_POINT('Ctrl Pts',(1.09986492944741,2.10000000001386,9.5103104176026));
#77159=CARTESIAN_POINT('Ctrl Pts',(1.0970064099584,2.10000000001386,9.49558664530564));
#77160=CARTESIAN_POINT('Ctrl Pts',(1.08515942970207,2.10000000001386,9.46742202035628));
#77161=CARTESIAN_POINT('Ctrl Pts',(1.07660754285019,2.10000000001387,9.45632598074318));
#77162=CARTESIAN_POINT('Ctrl Pts',(1.05826102775228,2.10000000001387,9.43763911093102));
#77163=CARTESIAN_POINT('Ctrl Pts',(1.04583977158587,2.10000000001387,9.42908030448567));
#77164=CARTESIAN_POINT('Ctrl Pts',(1.01700990292886,2.10000000001387,9.41681005498998));
#77165=CARTESIAN_POINT('Ctrl Pts',(1.00311689049416,2.10000000001388,9.41499747796185));
#77166=CARTESIAN_POINT('Ctrl Pts',(0.977374576676416,2.10000000001388,9.41483734650305));
#77167=CARTESIAN_POINT('Ctrl Pts',(0.963017667221115,2.1000000000139,9.41753459916267));
#77168=CARTESIAN_POINT('Ctrl Pts',(0.938227536233048,2.1000000000139,9.42720438574357));
#77169=CARTESIAN_POINT('Ctrl Pts',(0.925632691761865,2.10000000001391,9.43421015995138));
#77170=CARTESIAN_POINT('Ctrl Pts',(0.90406812267464,2.10000000001391,9.45502871027269));
#77171=CARTESIAN_POINT('Ctrl Pts',(0.896008094926436,2.10000000001392,9.46655439418273));
#77172=CARTESIAN_POINT('Ctrl Pts',(0.884146571951397,2.10000000001392,9.49234046373837));
#77173=CARTESIAN_POINT('Ctrl Pts',(0.88058305209276,2.10000000001394,9.50675642080951));
#77174=CARTESIAN_POINT('Ctrl Pts',(0.880021960842162,2.10000000001394,9.52254283629876));
#77175=CARTESIAN_POINT('Ctrl Pts',(0.88,2.1,9.52377137958177));
#77176=CARTESIAN_POINT('Ctrl Pts',(0.88,2.1,9.525));
#77177=CARTESIAN_POINT('',(-1.09265261173395,2.09796323888708,12.2355247810852));
#77178=CARTESIAN_POINT('Ctrl Pts',(0.88,2.1,9.525));
#77179=CARTESIAN_POINT('Ctrl Pts',(0.879914606625585,2.17110785049955,9.52865476385635));
#77180=CARTESIAN_POINT('Ctrl Pts',(0.863232117186907,2.3095104036224,9.53591397312323));
#77181=CARTESIAN_POINT('Ctrl Pts',(0.7646146646842,2.57432753790838,9.55048599717583));
#77182=CARTESIAN_POINT('Ctrl Pts',(0.52875066403414,2.8457083400553,9.56867094599734));
#77183=CARTESIAN_POINT('Ctrl Pts',(0.127238756664634,3.00552936974926,9.59051359518968));
#77184=CARTESIAN_POINT('Ctrl Pts',(-0.302716205619033,2.96306288294985,
9.61235380295566));
#77185=CARTESIAN_POINT('Ctrl Pts',(-0.665427657999688,2.72799341501097,
9.63420407641812));
#77186=CARTESIAN_POINT('Ctrl Pts',(-0.879826065415376,2.3524940033895,9.65606121698024));
#77187=CARTESIAN_POINT('Ctrl Pts',(-0.89799221853441,1.92029343459682,9.67792905414005));
#77188=CARTESIAN_POINT('Ctrl Pts',(-0.715657796510551,1.52775201761214,
9.69980826165769));
#77189=CARTESIAN_POINT('Ctrl Pts',(-0.37329244035757,1.26252484692041,9.72170089413125));
#77190=CARTESIAN_POINT('Ctrl Pts',(0.0529042162174613,1.18397194405211,
9.7436083723133));
#77191=CARTESIAN_POINT('Ctrl Pts',(0.467926525737336,1.30987826775351,9.76553239226868));
#77192=CARTESIAN_POINT('Ctrl Pts',(0.77911594458734,1.61250328722602,9.78747453406851));
#77193=CARTESIAN_POINT('Ctrl Pts',(0.916833254715888,2.02450810034898,9.8094364412056));
#77194=CARTESIAN_POINT('Ctrl Pts',(0.84999015619955,2.45432327019144,9.83141968646686));
#77195=CARTESIAN_POINT('Ctrl Pts',(0.593134887517594,2.80556810401153,9.85342584950507));
#77196=CARTESIAN_POINT('Ctrl Pts',(0.159785468035136,3.02235194398505,9.87790429996245));
#77197=CARTESIAN_POINT('Ctrl Pts',(-0.382738476891779,2.97204316801605,
9.90486768286448));
#77198=CARTESIAN_POINT('Ctrl Pts',(-0.827943575417754,2.57464859578558,
9.93433214776037));
#77199=CARTESIAN_POINT('Ctrl Pts',(-0.928540642244484,2.0879125901631,9.95893043030863));
#77200=CARTESIAN_POINT('Ctrl Pts',(-0.82506221727755,1.71823863855703,9.97863755083128));
#77201=CARTESIAN_POINT('Ctrl Pts',(-0.665238898770628,1.47861418311032,
9.99343255715118));
#77202=CARTESIAN_POINT('Ctrl Pts',(-0.438025190317537,1.3012081221325,10.0082426633322));
#77203=CARTESIAN_POINT('Ctrl Pts',(-0.0759140953759721,1.16989403941721,
10.0280101634631));
#77204=CARTESIAN_POINT('Ctrl Pts',(0.353590617267489,1.22647296601624,10.0494595111079));
#77205=CARTESIAN_POINT('Ctrl Pts',(0.71282299611785,1.50640456177768,10.0726022736917));
#77206=CARTESIAN_POINT('Ctrl Pts',(0.895311256816217,1.85157831854142,10.0924697020734));
#77207=CARTESIAN_POINT('Ctrl Pts',(0.917661293713379,2.20976194577009,10.1107106042816));
#77208=CARTESIAN_POINT('Ctrl Pts',(0.819212469046223,2.51761130734418,10.127317066638));
#77209=CARTESIAN_POINT('Ctrl Pts',(0.591924394917487,2.83289082559773,10.1472698428113));
#77210=CARTESIAN_POINT('Ctrl Pts',(0.141288805504938,3.06103897732418,10.172258699084));
#77211=CARTESIAN_POINT('Ctrl Pts',(-0.458527011040082,2.95925151709148,
10.2023249565719));
#77212=CARTESIAN_POINT('Ctrl Pts',(-0.88162766536303,2.52027411449529,10.2324736532743));
#77213=CARTESIAN_POINT('Ctrl Pts',(-0.961653185964405,1.91393657438503,
10.2627077273853));
#77214=CARTESIAN_POINT('Ctrl Pts',(-0.665231767857691,1.37715957803001,
10.2930297792945));
#77215=CARTESIAN_POINT('Ctrl Pts',(-0.105988685338195,1.12026073865136,
10.3234425669733));
#77216=CARTESIAN_POINT('Ctrl Pts',(0.430538820721984,1.23255710504194,10.3505590141325));
#77217=CARTESIAN_POINT('Ctrl Pts',(0.777157271318668,1.54704609431923,10.3743479205533));
#77218=CARTESIAN_POINT('Ctrl Pts',(0.937973646848606,1.91510656924282,10.3947816504623));
#77219=CARTESIAN_POINT('Ctrl Pts',(0.932931736507626,2.31778957988939,10.4152592321293));
#77220=CARTESIAN_POINT('Ctrl Pts',(0.762578582228501,2.68366310973811,10.4357813746755));
#77221=CARTESIAN_POINT('Ctrl Pts',(0.455963235969408,2.94715653506223,10.4563486739678));
#77222=CARTESIAN_POINT('Ctrl Pts',(0.00240142086611935,3.08166579400621,
10.480397254692));
#77223=CARTESIAN_POINT('Ctrl Pts',(-0.538455390507358,2.94820992747045,
10.5079586157699));
#77224=CARTESIAN_POINT('Ctrl Pts',(-0.940666416691817,2.46401744657124,
10.5390713811047));
#77225=CARTESIAN_POINT('Ctrl Pts',(-0.976029443563649,1.83335883304997,
10.5702921359498));
#77226=CARTESIAN_POINT('Ctrl Pts',(-0.629306856593687,1.30317046301086,
10.6016225477596));
#77227=CARTESIAN_POINT('Ctrl Pts',(-0.0328763589810331,1.08144514613719,
10.6330641573791));
#77228=CARTESIAN_POINT('Ctrl Pts',(0.511901871764286,1.23876013099839,10.6611123163153));
#77229=CARTESIAN_POINT('Ctrl Pts',(0.845208777494887,1.59002857501027,10.6857282761483));
#77230=CARTESIAN_POINT('Ctrl Pts',(0.959937391714928,1.91692164410815,10.7033535735637));
#77231=CARTESIAN_POINT('Ctrl Pts',(0.964709509971458,2.19002072343591,10.7174794574177));
#77232=CARTESIAN_POINT('Ctrl Pts',(0.903969607200192,2.50338072207659,10.7339796596208));
#77233=CARTESIAN_POINT('Ctrl Pts',(0.708976511873778,2.79903473649909,10.7516978643424));
#77234=CARTESIAN_POINT('Ctrl Pts',(0.359111666410103,3.02058677865832,10.7730116718645));
#77235=CARTESIAN_POINT('Ctrl Pts',(-0.0055195068732309,3.09939687665217,
10.7919958841582));
#77236=CARTESIAN_POINT('Ctrl Pts',(-0.417331250225881,3.01093271757532,
10.8134054790171));
#77237=CARTESIAN_POINT('Ctrl Pts',(-0.756608961158023,2.76032613000462,
10.8348676292604));
#77238=CARTESIAN_POINT('Ctrl Pts',(-0.998865593098056,2.33000290793379,
10.8599683150449));
#77239=CARTESIAN_POINT('Ctrl Pts',(-0.988791187924089,1.74845036869023,
10.8887429491342));
#77240=CARTESIAN_POINT('Ctrl Pts',(-0.588714669350558,1.22669384301482,
10.9212338011637));
#77241=CARTESIAN_POINT('Ctrl Pts',(0.044909234496707,1.04388405761621,10.9538443040117));
#77242=CARTESIAN_POINT('Ctrl Pts',(0.665762350574508,1.27382859359802,10.9865746011287));
#77243=CARTESIAN_POINT('Ctrl Pts',(1.02994927065475,1.82963242200099,11.0194247010519));
#77244=CARTESIAN_POINT('Ctrl Pts',(0.99292771913683,2.49532007970257,11.0523944801788));
#77245=CARTESIAN_POINT('Ctrl Pts',(0.566047404042377,3.01118540039736,11.0854836852924));
#77246=CARTESIAN_POINT('Ctrl Pts',(-0.0131656805453273,3.1545072720966,
11.1150021335127));
#77247=CARTESIAN_POINT('Ctrl Pts',(-0.501834747536299,3.00971245930524,
11.1409075995603));
#77248=CARTESIAN_POINT('Ctrl Pts',(-0.833654637909307,2.72466132918788,
11.1631647757637));
#77249=CARTESIAN_POINT('Ctrl Pts',(-1.01904932840502,2.32688792491809,11.1854742337572));
#77250=CARTESIAN_POINT('Ctrl Pts',(-1.0247320303861,1.8873087550975,11.2078357472338));
#77251=CARTESIAN_POINT('Ctrl Pts',(-0.848433071641297,1.48323440703255,
11.2302490424206));
#77252=CARTESIAN_POINT('Ctrl Pts',(-0.5209916303453,1.18686010809674,11.2527138516101));
#77253=CARTESIAN_POINT('Ctrl Pts',(-0.0994474829318688,1.05086828612434,
11.2752298585268));
#77254=CARTESIAN_POINT('Ctrl Pts',(0.341286571712092,1.10081439784123,11.297796723956));
#77255=CARTESIAN_POINT('Ctrl Pts',(0.787934060544661,1.36522529701193,11.3241836591263));
#77256=CARTESIAN_POINT('Ctrl Pts',(1.08440822726537,1.89981767692546,11.3544236935599));
#77257=CARTESIAN_POINT('Ctrl Pts',(0.99437189083192,2.58466520846377,11.3885550724356));
#77258=CARTESIAN_POINT('Ctrl Pts',(0.51422832678732,3.08343949927552,11.4227963300144));
#77259=CARTESIAN_POINT('Ctrl Pts',(-0.170956362315584,3.20042729316684,
11.4571457685877));
#77260=CARTESIAN_POINT('Ctrl Pts',(-0.792809143568463,2.88603885152724,
11.49160167588));
#77261=CARTESIAN_POINT('Ctrl Pts',(-1.10815562220614,2.26212033857722,11.5261621918766));
#77262=CARTESIAN_POINT('Ctrl Pts',(-0.990980784814367,1.57098681332194,
11.5608252913622));
#77263=CARTESIAN_POINT('Ctrl Pts',(-0.484736723033935,1.08260154598769,
11.5955889188738));
#77264=CARTESIAN_POINT('Ctrl Pts',(0.214307763377102,0.991032096532327,
11.6304507824074));
#77265=CARTESIAN_POINT('Ctrl Pts',(0.833298379906107,1.33271197734595,11.6654086518246));
#77266=CARTESIAN_POINT('Ctrl Pts',(1.12908711130714,1.97705558535849,11.7004600148669));
#77267=CARTESIAN_POINT('Ctrl Pts',(0.984170425255086,2.67277304384029,11.7356024461146));
#77268=CARTESIAN_POINT('Ctrl Pts',(0.452808643636702,3.14802102155422,11.7708333087139));
#77269=CARTESIAN_POINT('Ctrl Pts',(-0.198836507924274,3.20872213800758,
11.8032068201948));
#77270=CARTESIAN_POINT('Ctrl Pts',(-0.720833985617695,2.9475724124579,11.8326976979388));
#77271=CARTESIAN_POINT('Ctrl Pts',(-1.03122512713103,2.52323917223077,11.8592848682016));
#77272=CARTESIAN_POINT('Ctrl Pts',(-1.11221371795246,2.00254397936835,11.8859162010712));
#77273=CARTESIAN_POINT('Ctrl Pts',(-0.944978677865563,1.50212478400673,
11.9125904181942));
#77274=CARTESIAN_POINT('Ctrl Pts',(-0.566096651435205,1.13364169683645,
11.9393062323883));
#77275=CARTESIAN_POINT('Ctrl Pts',(-0.0596069971212731,0.97996909355213,
11.966062281935));
#77276=CARTESIAN_POINT('Ctrl Pts',(0.461675051948685,1.07603593590851,11.9928572469173));
#77277=CARTESIAN_POINT('Ctrl Pts',(0.88129231323125,1.40110770643291,12.0196896905075));
#77278=CARTESIAN_POINT('Ctrl Pts',(1.10519737818586,1.88315811002375,12.0465583931276));
#77279=CARTESIAN_POINT('Ctrl Pts',(1.08283365883886,2.41488670097258,12.0734615789711));
#77280=CARTESIAN_POINT('Ctrl Pts',(0.818591168747924,2.87760074176854,12.100398642491));
#77281=CARTESIAN_POINT('Ctrl Pts',(0.370893737846914,3.16774776724325,12.1273662612715));
#77282=CARTESIAN_POINT('Ctrl Pts',(-0.160578831483255,3.22009488317826,
12.154367120808));
#77283=CARTESIAN_POINT('Ctrl Pts',(-0.657438304412148,3.02243699025829,
12.181390412703));
#77284=CARTESIAN_POINT('Ctrl Pts',(-0.949764066307816,2.68573447988004,
12.2039450357004));
#77285=CARTESIAN_POINT('Ctrl Pts',(-1.07182425162092,2.35796849387404,12.2219800536891));
#77286=CARTESIAN_POINT('Ctrl Pts',(-1.09256785760649,2.18550272007321,12.2310256553714));
#77287=CARTESIAN_POINT('Ctrl Pts',(-1.09265261173395,2.09796323888708,12.2355247810852));
#77288=CARTESIAN_POINT('Ctrl Pts',(-1.09265261173395,2.09796323888708,12.2355247810852));
#77289=CARTESIAN_POINT('Ctrl Pts',(-1.09209725849391,2.09780929004959,12.2340885660349));
#77290=CARTESIAN_POINT('Ctrl Pts',(-1.09150942605389,2.09765599988943,12.2326649833975));
#77291=CARTESIAN_POINT('Ctrl Pts',(-1.08503237448485,2.09606086603517,12.217918236082));
#77292=CARTESIAN_POINT('Ctrl Pts',(-1.07637147919497,2.09469021271178,12.2058229006299));
#77293=CARTESIAN_POINT('Ctrl Pts',(-1.05589660811711,2.09236330772606,12.1863633679792));
#77294=CARTESIAN_POINT('Ctrl Pts',(-1.04427559806097,2.09138110303581,12.1787037088208));
#77295=CARTESIAN_POINT('Ctrl Pts',(-1.01685371830238,2.08974317821197,12.1674274156938));
#77296=CARTESIAN_POINT('Ctrl Pts',(-1.00269310527362,2.08929246375968,12.1655556665659));
#77297=CARTESIAN_POINT('Ctrl Pts',(-0.976082721926214,2.08880858272302,
12.1656694650394));
#77298=CARTESIAN_POINT('Ctrl Pts',(-0.961674722252946,2.08881998593982,
12.1684652160567));
#77299=CARTESIAN_POINT('Ctrl Pts',(-0.935145584204836,2.089393532376,12.1791388039753));
#77300=CARTESIAN_POINT('Ctrl Pts',(-0.923377726165856,2.08994242930189,
12.1868184150991));
#77301=CARTESIAN_POINT('Ctrl Pts',(-0.902773358098951,2.09158615536369,
12.2070916862902));
#77302=CARTESIAN_POINT('Ctrl Pts',(-0.894359321703738,2.09266703294608,
12.2194671888421));
#77303=CARTESIAN_POINT('Ctrl Pts',(-0.884085346464909,2.09486938130549,
12.2434042584418));
#77304=CARTESIAN_POINT('Ctrl Pts',(-0.880278658103152,2.09611450652452,
12.2565647862241));
#77305=CARTESIAN_POINT('Ctrl Pts',(-0.879499381119838,2.0990850140734,12.2864166942923));
#77306=CARTESIAN_POINT('Ctrl Pts',(-0.882184130880262,2.10058766003656,
12.3009443552539));
#77307=CARTESIAN_POINT('Ctrl Pts',(-0.892745023046883,2.10349559053314,
12.3280597480034));
#77308=CARTESIAN_POINT('Ctrl Pts',(-0.900696465100613,2.10490739378147,
12.3406986555977));
#77309=CARTESIAN_POINT('Ctrl Pts',(-0.921859448736967,2.10748987243997,
12.3625860027947));
#77310=CARTESIAN_POINT('Ctrl Pts',(-0.93382210431347,2.10843536774309,12.3698149566619));
#77311=CARTESIAN_POINT('Ctrl Pts',(-0.957649249474271,2.10995464694397,
12.3805737978547));
#77312=CARTESIAN_POINT('Ctrl Pts',(-0.972312296243169,2.11057609115668,
12.384059431092));
#77313=CARTESIAN_POINT('Ctrl Pts',(-1.00361986077531,2.11126293040044,12.3851010665202));
#77314=CARTESIAN_POINT('Ctrl Pts',(-1.0172353688322,2.11118600372854,12.3817975452729));
#77315=CARTESIAN_POINT('Ctrl Pts',(-1.04131570492226,2.11072528877995,12.3727081273419));
#77316=CARTESIAN_POINT('Ctrl Pts',(-1.05374570140234,2.11019113143425,12.3650526793176));
#77317=CARTESIAN_POINT('Ctrl Pts',(-1.0734098354843,2.10877015968504,12.3471820879167));
#77318=CARTESIAN_POINT('Ctrl Pts',(-1.08264928283733,2.10784001388133,12.3361603629656));
#77319=CARTESIAN_POINT('Ctrl Pts',(-1.095302396531,2.10536967950763,12.3091004509308));
#77320=CARTESIAN_POINT('Ctrl Pts',(-1.09868788747203,2.10407385649719,12.2955113107553));
#77321=CARTESIAN_POINT('Ctrl Pts',(-1.10050339267094,2.10128901138116,12.2673232691602));
#77322=CARTESIAN_POINT('Ctrl Pts',(-1.09865549775466,2.09978891927082,12.252665387318));
#77323=CARTESIAN_POINT('Ctrl Pts',(-1.09351390934533,2.09820808595437,12.2378130887736));
#77324=CARTESIAN_POINT('Ctrl Pts',(-1.09309352137022,2.09808546294386,12.2366650302271));
#77325=CARTESIAN_POINT('Ctrl Pts',(-1.09265261173395,2.09796323888708,12.2355247810852));
#77326=CARTESIAN_POINT('Origin',(-0.990000000000001,2.10000000000001,12.275));
#77327=CARTESIAN_POINT('Origin',(0.99,2.1,9.525));
#85757=UNCERTAINTY_MEASURE_WITH_UNIT(LENGTH_MEASURE(0.001),#85790,
'DISTANCE_ACCURACY_VALUE',
'Maximum model space distance between geometric entities at asserted c
onnectivities');
#85769=UNCERTAINTY_MEASURE_WITH_UNIT(LENGTH_MEASURE(0.001),#85790,
'DISTANCE_ACCURACY_VALUE',
'Maximum model space distance between geometric entities at asserted c
onnectivities');
#85777=(
GEOMETRIC_REPRESENTATION_CONTEXT(3)
GLOBAL_UNCERTAINTY_ASSIGNED_CONTEXT((#85757))
GLOBAL_UNIT_ASSIGNED_CONTEXT((#85790,#85792,#85793))
REPRESENTATION_CONTEXT('','3D')
);
#85789=(
GEOMETRIC_REPRESENTATION_CONTEXT(3)
GLOBAL_UNCERTAINTY_ASSIGNED_CONTEXT((#85769))
GLOBAL_UNIT_ASSIGNED_CONTEXT((#85790,#85792,#85793))
REPRESENTATION_CONTEXT('','3D')
);
#85790=(
LENGTH_UNIT()
NAMED_UNIT(*)
SI_UNIT(.CENTI.,.METRE.)
);
#85792=(
NAMED_UNIT(*)
PLANE_ANGLE_UNIT()
SI_UNIT($,.RADIAN.)
);
#85793=(
NAMED_UNIT(*)
SI_UNIT($,.STERADIAN.)
SOLID_ANGLE_UNIT()
);
#85801=SHAPE_DEFINITION_REPRESENTATION(#85820,#85869);
#85820=PRODUCT_DEFINITION_SHAPE('',$,#85889);
#85869=SHAPE_REPRESENTATION('',(#10562),#85777);
#85881=PRODUCT_DEFINITION_CONTEXT('part definition',#85940,'design');
#85889=PRODUCT_DEFINITION('Preload Compression Spring d2.2',
'Preload Compression Spring d2.2',#85908,#85881);
#85908=PRODUCT_DEFINITION_FORMATION('',$,#85949);
#85940=APPLICATION_CONTEXT(
'Core Data for Automotive Mechanical Design Process');
#85941=PRODUCT_CONTEXT('part definition',#85940,'mechanical');
#85949=PRODUCT('Preload Compression Spring d2.2',
'Preload Compression Spring d2.2',$,(#85941));
#85968=PRESENTATION_STYLE_ASSIGNMENT((#85986));
#85986=SURFACE_STYLE_USAGE(.BOTH.,#86004);
#86004=SURFACE_SIDE_STYLE('',(#86022));
#86022=SURFACE_STYLE_FILL_AREA(#86040);
#86040=FILL_AREA_STYLE('Opaque(38,38,41)',(#86058));
#86058=FILL_AREA_STYLE_COLOUR('Opaque(38,38,41)',#86076);
#86076=COLOUR_RGB('Opaque(38,38,41)', 0.66274510, 0.83137255, 0.94901961);
ENDSEC;
END-ISO-10303-21;
